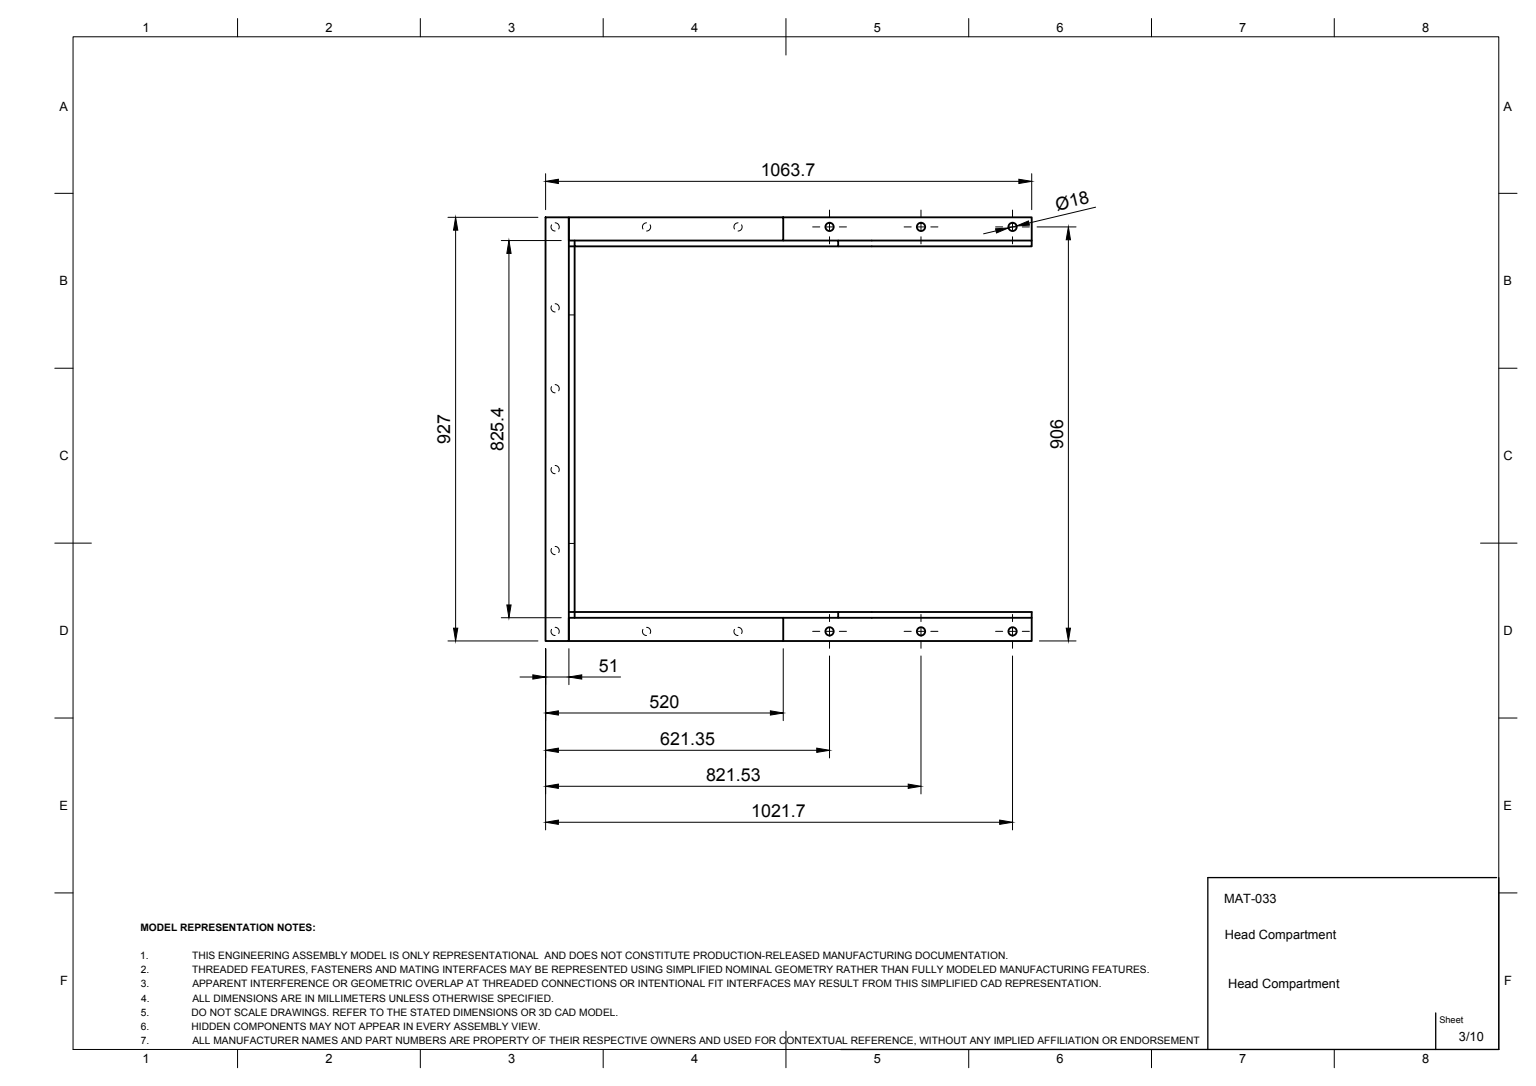
ISO-10303-21;
HEADER;
/* Generated by software containing ST-Developer
 * from STEP Tools, Inc. (www.steptools.com) 
 */

FILE_DESCRIPTION(
/* description */ ('STEP AP214'),
/* implementation_level */ '2;1');

FILE_NAME(
/* name */ 'Head Compartment.step',
/* time_stamp */ '2026-11-14T07:13:32-08:00',
/* author */ (''),
/* organization */ (''),
/* preprocessor_version */ 'ST-DEVELOPER v20.2',
/* originating_system */ 'Autodesk Translation Framework v15.17.0.0',
/* authorisation */ '');

FILE_SCHEMA (('AUTOMOTIVE_DESIGN { 1 0 10303 214 3 1 1 }'));
ENDSEC;

DATA;
#10=MECHANICAL_DESIGN_GEOMETRIC_PRESENTATION_REPRESENTATION('',(#1291,#1292,#1293,#1294,#1295,#1296,#1297,#1298,#1299),#32903);
#672=SHAPE_REPRESENTATION_RELATIONSHIP('SRR','None',#33013,#686);
#686=ADVANCED_BREP_SHAPE_REPRESENTATION('',(#1380,#1381,#1382,#1383,#1384,
#1385,#1386,#1387,#1388),#32888);
#700=CIRCLE('',#15798,75.0000000000001);
#701=CIRCLE('',#15799,75.0000000000001);
#702=CIRCLE('',#15808,75.0000000000001);
#703=CIRCLE('',#15809,75.0000000000001);
#704=CIRCLE('',#15816,8.99999999999998);
#705=CIRCLE('',#15817,8.99999999999998);
#706=CIRCLE('',#15819,8.99999999999998);
#707=CIRCLE('',#15820,8.99999999999998);
#708=CIRCLE('',#15822,8.99999999999998);
#709=CIRCLE('',#15823,8.99999999999998);
#710=CIRCLE('',#15825,8.99999999999998);
#711=CIRCLE('',#15826,8.99999999999998);
#712=CIRCLE('',#15828,8.99999999999998);
#713=CIRCLE('',#15829,8.99999999999998);
#714=CIRCLE('',#15831,8.99999999999998);
#715=CIRCLE('',#15832,8.99999999999998);
#716=CIRCLE('',#15840,8.99999999999998);
#717=CIRCLE('',#15841,8.99999999999998);
#718=CIRCLE('',#15843,9.00000000000001);
#719=CIRCLE('',#15844,9.00000000000001);
#720=CIRCLE('',#15846,9.00000000000001);
#721=CIRCLE('',#15847,9.00000000000001);
#722=CIRCLE('',#15849,9.00000000000001);
#723=CIRCLE('',#15850,9.00000000000001);
#724=CIRCLE('',#15852,9.00000000000001);
#725=CIRCLE('',#15853,9.00000000000001);
#726=CIRCLE('',#15861,8.99999999999998);
#727=CIRCLE('',#15862,8.99999999999998);
#728=CIRCLE('',#15864,9.00000000000001);
#729=CIRCLE('',#15865,9.00000000000001);
#730=CIRCLE('',#15867,9.00000000000001);
#731=CIRCLE('',#15868,9.00000000000001);
#732=CIRCLE('',#15870,9.00000000000001);
#733=CIRCLE('',#15871,9.00000000000001);
#734=CIRCLE('',#15873,9.00000000000001);
#735=CIRCLE('',#15874,9.00000000000001);
#1081=CYLINDRICAL_SURFACE('',#15797,75.0000000000001);
#1082=CYLINDRICAL_SURFACE('',#15807,75.0000000000001);
#1083=CYLINDRICAL_SURFACE('',#15815,8.99999999999998);
#1084=CYLINDRICAL_SURFACE('',#15818,8.99999999999998);
#1085=CYLINDRICAL_SURFACE('',#15821,8.99999999999998);
#1086=CYLINDRICAL_SURFACE('',#15824,8.99999999999998);
#1087=CYLINDRICAL_SURFACE('',#15827,8.99999999999998);
#1088=CYLINDRICAL_SURFACE('',#15830,8.99999999999998);
#1089=CYLINDRICAL_SURFACE('',#15839,8.99999999999998);
#1090=CYLINDRICAL_SURFACE('',#15842,9.00000000000001);
#1091=CYLINDRICAL_SURFACE('',#15845,9.00000000000001);
#1092=CYLINDRICAL_SURFACE('',#15848,9.00000000000001);
#1093=CYLINDRICAL_SURFACE('',#15851,9.00000000000001);
#1094=CYLINDRICAL_SURFACE('',#15860,8.99999999999998);
#1095=CYLINDRICAL_SURFACE('',#15863,9.00000000000001);
#1096=CYLINDRICAL_SURFACE('',#15866,9.00000000000001);
#1097=CYLINDRICAL_SURFACE('',#15869,9.00000000000001);
#1098=CYLINDRICAL_SURFACE('',#15872,9.00000000000001);
#1291=STYLED_ITEM('',(#33097),#1380);
#1292=STYLED_ITEM('',(#33097),#1381);
#1293=STYLED_ITEM('',(#33097),#1382);
#1294=STYLED_ITEM('',(#33097),#1383);
#1295=STYLED_ITEM('',(#33097),#1384);
#1296=STYLED_ITEM('',(#33097),#1385);
#1297=STYLED_ITEM('',(#33097),#1386);
#1298=STYLED_ITEM('',(#33097),#1387);
#1299=STYLED_ITEM('',(#33097),#1388);
#1380=MANIFOLD_SOLID_BREP('Body1',#15539);
#1381=MANIFOLD_SOLID_BREP('Body2',#15540);
#1382=MANIFOLD_SOLID_BREP('Body3',#15541);
#1383=MANIFOLD_SOLID_BREP('Body4',#15542);
#1384=MANIFOLD_SOLID_BREP('Body5',#15543);
#1385=MANIFOLD_SOLID_BREP('Body6',#15544);
#1386=MANIFOLD_SOLID_BREP('Body7',#15545);
#1387=MANIFOLD_SOLID_BREP('Body8',#15546);
#1388=MANIFOLD_SOLID_BREP('Body9',#15547);
#1469=FACE_BOUND('',#2576,.T.);
#1470=FACE_BOUND('',#2578,.T.);
#1471=FACE_BOUND('',#2606,.T.);
#1472=FACE_BOUND('',#2607,.T.);
#1473=FACE_BOUND('',#2608,.T.);
#1474=FACE_BOUND('',#2609,.T.);
#1475=FACE_BOUND('',#2610,.T.);
#1476=FACE_BOUND('',#2611,.T.);
#1477=FACE_BOUND('',#2613,.T.);
#1478=FACE_BOUND('',#2614,.T.);
#1479=FACE_BOUND('',#2615,.T.);
#1480=FACE_BOUND('',#2616,.T.);
#1481=FACE_BOUND('',#2617,.T.);
#1482=FACE_BOUND('',#2618,.T.);
#1483=FACE_BOUND('',#2633,.T.);
#1484=FACE_BOUND('',#2634,.T.);
#1485=FACE_BOUND('',#2635,.T.);
#1486=FACE_BOUND('',#2636,.T.);
#1487=FACE_BOUND('',#2637,.T.);
#1488=FACE_BOUND('',#2639,.T.);
#1489=FACE_BOUND('',#2640,.T.);
#1490=FACE_BOUND('',#2641,.T.);
#1491=FACE_BOUND('',#2642,.T.);
#1492=FACE_BOUND('',#2643,.T.);
#1493=FACE_BOUND('',#2654,.T.);
#1494=FACE_BOUND('',#2655,.T.);
#1495=FACE_BOUND('',#2656,.T.);
#1496=FACE_BOUND('',#2657,.T.);
#1497=FACE_BOUND('',#2658,.T.);
#1498=FACE_BOUND('',#2660,.T.);
#1499=FACE_BOUND('',#2661,.T.);
#1500=FACE_BOUND('',#2662,.T.);
#1501=FACE_BOUND('',#2663,.T.);
#1502=FACE_BOUND('',#2664,.T.);
#1676=FACE_OUTER_BOUND('',#2571,.T.);
#1677=FACE_OUTER_BOUND('',#2572,.T.);
#1678=FACE_OUTER_BOUND('',#2573,.T.);
#1679=FACE_OUTER_BOUND('',#2574,.T.);
#1680=FACE_OUTER_BOUND('',#2575,.T.);
#1681=FACE_OUTER_BOUND('',#2577,.T.);
#1682=FACE_OUTER_BOUND('',#2579,.T.);
#1683=FACE_OUTER_BOUND('',#2580,.T.);
#1684=FACE_OUTER_BOUND('',#2581,.T.);
#1685=FACE_OUTER_BOUND('',#2582,.T.);
#1686=FACE_OUTER_BOUND('',#2583,.T.);
#1687=FACE_OUTER_BOUND('',#2584,.T.);
#1688=FACE_OUTER_BOUND('',#2585,.T.);
#1689=FACE_OUTER_BOUND('',#2586,.T.);
#1690=FACE_OUTER_BOUND('',#2587,.T.);
#1691=FACE_OUTER_BOUND('',#2588,.T.);
#1692=FACE_OUTER_BOUND('',#2589,.T.);
#1693=FACE_OUTER_BOUND('',#2590,.T.);
#1694=FACE_OUTER_BOUND('',#2591,.T.);
#1695=FACE_OUTER_BOUND('',#2592,.T.);
#1696=FACE_OUTER_BOUND('',#2593,.T.);
#1697=FACE_OUTER_BOUND('',#2594,.T.);
#1698=FACE_OUTER_BOUND('',#2595,.T.);
#1699=FACE_OUTER_BOUND('',#2596,.T.);
#1700=FACE_OUTER_BOUND('',#2597,.T.);
#1701=FACE_OUTER_BOUND('',#2598,.T.);
#1702=FACE_OUTER_BOUND('',#2599,.T.);
#1703=FACE_OUTER_BOUND('',#2600,.T.);
#1704=FACE_OUTER_BOUND('',#2601,.T.);
#1705=FACE_OUTER_BOUND('',#2602,.T.);
#1706=FACE_OUTER_BOUND('',#2603,.T.);
#1707=FACE_OUTER_BOUND('',#2604,.T.);
#1708=FACE_OUTER_BOUND('',#2605,.T.);
#1709=FACE_OUTER_BOUND('',#2612,.T.);
#1710=FACE_OUTER_BOUND('',#2619,.T.);
#1711=FACE_OUTER_BOUND('',#2620,.T.);
#1712=FACE_OUTER_BOUND('',#2621,.T.);
#1713=FACE_OUTER_BOUND('',#2622,.T.);
#1714=FACE_OUTER_BOUND('',#2623,.T.);
#1715=FACE_OUTER_BOUND('',#2624,.T.);
#1716=FACE_OUTER_BOUND('',#2625,.T.);
#1717=FACE_OUTER_BOUND('',#2626,.T.);
#1718=FACE_OUTER_BOUND('',#2627,.T.);
#1719=FACE_OUTER_BOUND('',#2628,.T.);
#1720=FACE_OUTER_BOUND('',#2629,.T.);
#1721=FACE_OUTER_BOUND('',#2630,.T.);
#1722=FACE_OUTER_BOUND('',#2631,.T.);
#1723=FACE_OUTER_BOUND('',#2632,.T.);
#1724=FACE_OUTER_BOUND('',#2638,.T.);
#1725=FACE_OUTER_BOUND('',#2644,.T.);
#1726=FACE_OUTER_BOUND('',#2645,.T.);
#1727=FACE_OUTER_BOUND('',#2646,.T.);
#1728=FACE_OUTER_BOUND('',#2647,.T.);
#1729=FACE_OUTER_BOUND('',#2648,.T.);
#1730=FACE_OUTER_BOUND('',#2649,.T.);
#1731=FACE_OUTER_BOUND('',#2650,.T.);
#1732=FACE_OUTER_BOUND('',#2651,.T.);
#1733=FACE_OUTER_BOUND('',#2652,.T.);
#1734=FACE_OUTER_BOUND('',#2653,.T.);
#1735=FACE_OUTER_BOUND('',#2659,.T.);
#1736=FACE_OUTER_BOUND('',#2665,.T.);
#1737=FACE_OUTER_BOUND('',#2666,.T.);
#1738=FACE_OUTER_BOUND('',#2667,.T.);
#1739=FACE_OUTER_BOUND('',#2668,.T.);
#1740=FACE_OUTER_BOUND('',#2669,.T.);
#1741=FACE_OUTER_BOUND('',#2670,.T.);
#1742=FACE_OUTER_BOUND('',#2671,.T.);
#1743=FACE_OUTER_BOUND('',#2672,.T.);
#1744=FACE_OUTER_BOUND('',#2673,.T.);
#1745=FACE_OUTER_BOUND('',#2674,.T.);
#1746=FACE_OUTER_BOUND('',#2675,.T.);
#1747=FACE_OUTER_BOUND('',#2676,.T.);
#1748=FACE_OUTER_BOUND('',#2677,.T.);
#1749=FACE_OUTER_BOUND('',#2678,.T.);
#1750=FACE_OUTER_BOUND('',#2679,.T.);
#1751=FACE_OUTER_BOUND('',#2680,.T.);
#1752=FACE_OUTER_BOUND('',#2681,.T.);
#1753=FACE_OUTER_BOUND('',#2682,.T.);
#2571=EDGE_LOOP('',(#9907,#9908,#9909,#9910));
#2572=EDGE_LOOP('',(#9911,#9912,#9913,#9914));
#2573=EDGE_LOOP('',(#9915,#9916,#9917,#9918));
#2574=EDGE_LOOP('',(#9919,#9920,#9921,#9922));
#2575=EDGE_LOOP('',(#9923,#9924,#9925,#9926));
#2576=EDGE_LOOP('',(#9927,#9928,#9929,#9930));
#2577=EDGE_LOOP('',(#9931,#9932,#9933,#9934));
#2578=EDGE_LOOP('',(#9935,#9936,#9937,#9938));
#2579=EDGE_LOOP('',(#9939,#9940,#9941,#9942));
#2580=EDGE_LOOP('',(#9943,#9944,#9945,#9946));
#2581=EDGE_LOOP('',(#9947,#9948,#9949,#9950));
#2582=EDGE_LOOP('',(#9951,#9952,#9953,#9954));
#2583=EDGE_LOOP('',(#9955,#9956,#9957,#9958));
#2584=EDGE_LOOP('',(#9959,#9960,#9961,#9962));
#2585=EDGE_LOOP('',(#9963,#9964,#9965,#9966));
#2586=EDGE_LOOP('',(#9967,#9968,#9969,#9970));
#2587=EDGE_LOOP('',(#9971,#9972,#9973,#9974));
#2588=EDGE_LOOP('',(#9975,#9976,#9977,#9978));
#2589=EDGE_LOOP('',(#9979,#9980,#9981,#9982,#9983,#9984));
#2590=EDGE_LOOP('',(#9985,#9986,#9987,#9988,#9989,#9990));
#2591=EDGE_LOOP('',(#9991,#9992,#9993,#9994));
#2592=EDGE_LOOP('',(#9995,#9996,#9997,#9998));
#2593=EDGE_LOOP('',(#9999,#10000,#10001,#10002));
#2594=EDGE_LOOP('',(#10003,#10004,#10005,#10006));
#2595=EDGE_LOOP('',(#10007,#10008,#10009,#10010));
#2596=EDGE_LOOP('',(#10011,#10012,#10013,#10014));
#2597=EDGE_LOOP('',(#10015,#10016,#10017,#10018,#10019,#10020));
#2598=EDGE_LOOP('',(#10021,#10022,#10023,#10024,#10025,#10026));
#2599=EDGE_LOOP('',(#10027,#10028,#10029,#10030));
#2600=EDGE_LOOP('',(#10031,#10032,#10033,#10034));
#2601=EDGE_LOOP('',(#10035,#10036,#10037,#10038));
#2602=EDGE_LOOP('',(#10039,#10040,#10041,#10042));
#2603=EDGE_LOOP('',(#10043,#10044,#10045,#10046));
#2604=EDGE_LOOP('',(#10047,#10048,#10049,#10050));
#2605=EDGE_LOOP('',(#10051,#10052,#10053,#10054));
#2606=EDGE_LOOP('',(#10055));
#2607=EDGE_LOOP('',(#10056));
#2608=EDGE_LOOP('',(#10057));
#2609=EDGE_LOOP('',(#10058));
#2610=EDGE_LOOP('',(#10059));
#2611=EDGE_LOOP('',(#10060));
#2612=EDGE_LOOP('',(#10061,#10062,#10063,#10064));
#2613=EDGE_LOOP('',(#10065));
#2614=EDGE_LOOP('',(#10066));
#2615=EDGE_LOOP('',(#10067));
#2616=EDGE_LOOP('',(#10068));
#2617=EDGE_LOOP('',(#10069));
#2618=EDGE_LOOP('',(#10070));
#2619=EDGE_LOOP('',(#10071,#10072,#10073,#10074));
#2620=EDGE_LOOP('',(#10075,#10076,#10077,#10078));
#2621=EDGE_LOOP('',(#10079,#10080,#10081,#10082));
#2622=EDGE_LOOP('',(#10083,#10084,#10085,#10086));
#2623=EDGE_LOOP('',(#10087,#10088,#10089,#10090));
#2624=EDGE_LOOP('',(#10091,#10092,#10093,#10094));
#2625=EDGE_LOOP('',(#10095,#10096,#10097,#10098));
#2626=EDGE_LOOP('',(#10099,#10100,#10101,#10102));
#2627=EDGE_LOOP('',(#10103,#10104,#10105,#10106));
#2628=EDGE_LOOP('',(#10107,#10108,#10109,#10110));
#2629=EDGE_LOOP('',(#10111,#10112,#10113,#10114));
#2630=EDGE_LOOP('',(#10115,#10116,#10117,#10118));
#2631=EDGE_LOOP('',(#10119,#10120,#10121,#10122));
#2632=EDGE_LOOP('',(#10123,#10124,#10125,#10126));
#2633=EDGE_LOOP('',(#10127));
#2634=EDGE_LOOP('',(#10128));
#2635=EDGE_LOOP('',(#10129));
#2636=EDGE_LOOP('',(#10130));
#2637=EDGE_LOOP('',(#10131));
#2638=EDGE_LOOP('',(#10132,#10133,#10134,#10135));
#2639=EDGE_LOOP('',(#10136));
#2640=EDGE_LOOP('',(#10137));
#2641=EDGE_LOOP('',(#10138));
#2642=EDGE_LOOP('',(#10139));
#2643=EDGE_LOOP('',(#10140));
#2644=EDGE_LOOP('',(#10141,#10142,#10143,#10144));
#2645=EDGE_LOOP('',(#10145,#10146,#10147,#10148));
#2646=EDGE_LOOP('',(#10149,#10150,#10151,#10152));
#2647=EDGE_LOOP('',(#10153,#10154,#10155,#10156));
#2648=EDGE_LOOP('',(#10157,#10158,#10159,#10160));
#2649=EDGE_LOOP('',(#10161,#10162,#10163,#10164));
#2650=EDGE_LOOP('',(#10165,#10166,#10167,#10168));
#2651=EDGE_LOOP('',(#10169,#10170,#10171,#10172));
#2652=EDGE_LOOP('',(#10173,#10174,#10175,#10176));
#2653=EDGE_LOOP('',(#10177,#10178,#10179,#10180));
#2654=EDGE_LOOP('',(#10181));
#2655=EDGE_LOOP('',(#10182));
#2656=EDGE_LOOP('',(#10183));
#2657=EDGE_LOOP('',(#10184));
#2658=EDGE_LOOP('',(#10185));
#2659=EDGE_LOOP('',(#10186,#10187,#10188,#10189));
#2660=EDGE_LOOP('',(#10190));
#2661=EDGE_LOOP('',(#10191));
#2662=EDGE_LOOP('',(#10192));
#2663=EDGE_LOOP('',(#10193));
#2664=EDGE_LOOP('',(#10194));
#2665=EDGE_LOOP('',(#10195,#10196,#10197,#10198));
#2666=EDGE_LOOP('',(#10199,#10200,#10201,#10202));
#2667=EDGE_LOOP('',(#10203,#10204,#10205,#10206));
#2668=EDGE_LOOP('',(#10207,#10208,#10209,#10210));
#2669=EDGE_LOOP('',(#10211,#10212,#10213,#10214));
#2670=EDGE_LOOP('',(#10215,#10216,#10217,#10218));
#2671=EDGE_LOOP('',(#10219,#10220,#10221,#10222));
#2672=EDGE_LOOP('',(#10223,#10224,#10225,#10226));
#2673=EDGE_LOOP('',(#10227,#10228,#10229,#10230));
#2674=EDGE_LOOP('',(#10231,#10232,#10233,#10234));
#2675=EDGE_LOOP('',(#10235,#10236,#10237,#10238));
#2676=EDGE_LOOP('',(#10239,#10240,#10241,#10242));
#2677=EDGE_LOOP('',(#10243,#10244,#10245,#10246));
#2678=EDGE_LOOP('',(#10247,#10248,#10249,#10250));
#2679=EDGE_LOOP('',(#10251,#10252,#10253,#10254));
#2680=EDGE_LOOP('',(#10255,#10256,#10257,#10258));
#2681=EDGE_LOOP('',(#10259,#10260,#10261,#10262));
#2682=EDGE_LOOP('',(#10263,#10264,#10265,#10266));
#3673=LINE('',#21314,#5077);
#3674=LINE('',#21316,#5078);
#3675=LINE('',#21318,#5079);
#3676=LINE('',#21319,#5080);
#3677=LINE('',#21322,#5081);
#3678=LINE('',#21324,#5082);
#3679=LINE('',#21325,#5083);
#3680=LINE('',#21328,#5084);
#3681=LINE('',#21330,#5085);
#3682=LINE('',#21331,#5086);
#3683=LINE('',#21333,#5087);
#3684=LINE('',#21334,#5088);
#3685=LINE('',#21338,#5089);
#3686=LINE('',#21340,#5090);
#3687=LINE('',#21342,#5091);
#3688=LINE('',#21343,#5092);
#3689=LINE('',#21347,#5093);
#3690=LINE('',#21349,#5094);
#3691=LINE('',#21351,#5095);
#3692=LINE('',#21352,#5096);
#3693=LINE('',#21354,#5097);
#3694=LINE('',#21355,#5098);
#3695=LINE('',#21357,#5099);
#3696=LINE('',#21359,#5100);
#3697=LINE('',#21364,#5101);
#3698=LINE('',#21366,#5102);
#3699=LINE('',#21368,#5103);
#3700=LINE('',#21369,#5104);
#3701=LINE('',#21372,#5105);
#3702=LINE('',#21374,#5106);
#3703=LINE('',#21375,#5107);
#3704=LINE('',#21380,#5108);
#3705=LINE('',#21384,#5109);
#3706=LINE('',#21386,#5110);
#3707=LINE('',#21387,#5111);
#3708=LINE('',#21390,#5112);
#3709=LINE('',#21392,#5113);
#3710=LINE('',#21393,#5114);
#3711=LINE('',#21395,#5115);
#3712=LINE('',#21396,#5116);
#3713=LINE('',#21402,#5117);
#3714=LINE('',#21404,#5118);
#3715=LINE('',#21406,#5119);
#3716=LINE('',#21407,#5120);
#3717=LINE('',#21410,#5121);
#3718=LINE('',#21412,#5122);
#3719=LINE('',#21413,#5123);
#3720=LINE('',#21419,#5124);
#3721=LINE('',#21422,#5125);
#3722=LINE('',#21424,#5126);
#3723=LINE('',#21425,#5127);
#3724=LINE('',#21428,#5128);
#3725=LINE('',#21430,#5129);
#3726=LINE('',#21431,#5130);
#3727=LINE('',#21433,#5131);
#3728=LINE('',#21434,#5132);
#3729=LINE('',#21441,#5133);
#3730=LINE('',#21447,#5134);
#3731=LINE('',#21453,#5135);
#3732=LINE('',#21459,#5136);
#3733=LINE('',#21465,#5137);
#3734=LINE('',#21471,#5138);
#3735=LINE('',#21476,#5139);
#3736=LINE('',#21478,#5140);
#3737=LINE('',#21480,#5141);
#3738=LINE('',#21481,#5142);
#3739=LINE('',#21485,#5143);
#3740=LINE('',#21487,#5144);
#3741=LINE('',#21489,#5145);
#3742=LINE('',#21490,#5146);
#3743=LINE('',#21492,#5147);
#3744=LINE('',#21493,#5148);
#3745=LINE('',#21495,#5149);
#3746=LINE('',#21497,#5150);
#3747=LINE('',#21503,#5151);
#3748=LINE('',#21509,#5152);
#3749=LINE('',#21515,#5153);
#3750=LINE('',#21521,#5154);
#3751=LINE('',#21527,#5155);
#3752=LINE('',#21532,#5156);
#3753=LINE('',#21534,#5157);
#3754=LINE('',#21536,#5158);
#3755=LINE('',#21537,#5159);
#3756=LINE('',#21540,#5160);
#3757=LINE('',#21542,#5161);
#3758=LINE('',#21543,#5162);
#3759=LINE('',#21546,#5163);
#3760=LINE('',#21548,#5164);
#3761=LINE('',#21549,#5165);
#3762=LINE('',#21551,#5166);
#3763=LINE('',#21552,#5167);
#3764=LINE('',#21559,#5168);
#3765=LINE('',#21565,#5169);
#3766=LINE('',#21571,#5170);
#3767=LINE('',#21577,#5171);
#3768=LINE('',#21583,#5172);
#3769=LINE('',#21588,#5173);
#3770=LINE('',#21590,#5174);
#3771=LINE('',#21592,#5175);
#3772=LINE('',#21593,#5176);
#3773=LINE('',#21596,#5177);
#3774=LINE('',#21598,#5178);
#3775=LINE('',#21599,#5179);
#3776=LINE('',#21602,#5180);
#3777=LINE('',#21604,#5181);
#3778=LINE('',#21605,#5182);
#3779=LINE('',#21607,#5183);
#3780=LINE('',#21608,#5184);
#3781=LINE('',#21614,#5185);
#3782=LINE('',#21616,#5186);
#3783=LINE('',#21618,#5187);
#3784=LINE('',#21619,#5188);
#3785=LINE('',#21622,#5189);
#3786=LINE('',#21624,#5190);
#3787=LINE('',#21625,#5191);
#3788=LINE('',#21628,#5192);
#3789=LINE('',#21630,#5193);
#3790=LINE('',#21631,#5194);
#3791=LINE('',#21633,#5195);
#3792=LINE('',#21634,#5196);
#3793=LINE('',#21640,#5197);
#3794=LINE('',#21642,#5198);
#3795=LINE('',#21644,#5199);
#3796=LINE('',#21645,#5200);
#3797=LINE('',#21648,#5201);
#3798=LINE('',#21650,#5202);
#3799=LINE('',#21651,#5203);
#3800=LINE('',#21654,#5204);
#3801=LINE('',#21656,#5205);
#3802=LINE('',#21657,#5206);
#3803=LINE('',#21659,#5207);
#3804=LINE('',#21660,#5208);
#3805=LINE('',#21666,#5209);
#3806=LINE('',#21668,#5210);
#3807=LINE('',#21670,#5211);
#3808=LINE('',#21671,#5212);
#3809=LINE('',#21674,#5213);
#3810=LINE('',#21676,#5214);
#3811=LINE('',#21677,#5215);
#3812=LINE('',#21680,#5216);
#3813=LINE('',#21682,#5217);
#3814=LINE('',#21683,#5218);
#3815=LINE('',#21685,#5219);
#3816=LINE('',#21686,#5220);
#5077=VECTOR('',#17163,1000.);
#5078=VECTOR('',#17164,1000.);
#5079=VECTOR('',#17165,1000.);
#5080=VECTOR('',#17166,1000.);
#5081=VECTOR('',#17169,1000.);
#5082=VECTOR('',#17170,1000.);
#5083=VECTOR('',#17171,1000.);
#5084=VECTOR('',#17174,1000.);
#5085=VECTOR('',#17175,1000.);
#5086=VECTOR('',#17176,1000.);
#5087=VECTOR('',#17179,1000.);
#5088=VECTOR('',#17180,1000.);
#5089=VECTOR('',#17183,1000.);
#5090=VECTOR('',#17184,1000.);
#5091=VECTOR('',#17185,1000.);
#5092=VECTOR('',#17186,1000.);
#5093=VECTOR('',#17189,1000.);
#5094=VECTOR('',#17190,1000.);
#5095=VECTOR('',#17191,1000.);
#5096=VECTOR('',#17192,1000.);
#5097=VECTOR('',#17195,1000.);
#5098=VECTOR('',#17196,1000.);
#5099=VECTOR('',#17199,1000.);
#5100=VECTOR('',#17202,1000.);
#5101=VECTOR('',#17207,1000.);
#5102=VECTOR('',#17208,1000.);
#5103=VECTOR('',#17209,1000.);
#5104=VECTOR('',#17210,1000.);
#5105=VECTOR('',#17213,1000.);
#5106=VECTOR('',#17214,1000.);
#5107=VECTOR('',#17215,1000.);
#5108=VECTOR('',#17220,1000.);
#5109=VECTOR('',#17225,1000.);
#5110=VECTOR('',#17226,1000.);
#5111=VECTOR('',#17227,1000.);
#5112=VECTOR('',#17230,1000.);
#5113=VECTOR('',#17231,1000.);
#5114=VECTOR('',#17232,1000.);
#5115=VECTOR('',#17235,1000.);
#5116=VECTOR('',#17236,1000.);
#5117=VECTOR('',#17243,1000.);
#5118=VECTOR('',#17244,1000.);
#5119=VECTOR('',#17245,1000.);
#5120=VECTOR('',#17246,1000.);
#5121=VECTOR('',#17249,1000.);
#5122=VECTOR('',#17250,1000.);
#5123=VECTOR('',#17251,1000.);
#5124=VECTOR('',#17258,1000.);
#5125=VECTOR('',#17261,1000.);
#5126=VECTOR('',#17262,1000.);
#5127=VECTOR('',#17263,1000.);
#5128=VECTOR('',#17266,1000.);
#5129=VECTOR('',#17267,1000.);
#5130=VECTOR('',#17268,1000.);
#5131=VECTOR('',#17271,1000.);
#5132=VECTOR('',#17272,1000.);
#5133=VECTOR('',#17281,8.99999999999998);
#5134=VECTOR('',#17288,8.99999999999998);
#5135=VECTOR('',#17295,8.99999999999998);
#5136=VECTOR('',#17302,8.99999999999998);
#5137=VECTOR('',#17309,8.99999999999998);
#5138=VECTOR('',#17316,8.99999999999998);
#5139=VECTOR('',#17321,1000.);
#5140=VECTOR('',#17322,1000.);
#5141=VECTOR('',#17323,1000.);
#5142=VECTOR('',#17324,1000.);
#5143=VECTOR('',#17327,1000.);
#5144=VECTOR('',#17328,1000.);
#5145=VECTOR('',#17329,1000.);
#5146=VECTOR('',#17330,1000.);
#5147=VECTOR('',#17333,1000.);
#5148=VECTOR('',#17334,1000.);
#5149=VECTOR('',#17337,1000.);
#5150=VECTOR('',#17340,1000.);
#5151=VECTOR('',#17347,8.99999999999998);
#5152=VECTOR('',#17354,9.00000000000001);
#5153=VECTOR('',#17361,9.00000000000001);
#5154=VECTOR('',#17368,9.00000000000001);
#5155=VECTOR('',#17375,9.00000000000001);
#5156=VECTOR('',#17380,1000.);
#5157=VECTOR('',#17381,1000.);
#5158=VECTOR('',#17382,1000.);
#5159=VECTOR('',#17383,1000.);
#5160=VECTOR('',#17386,1000.);
#5161=VECTOR('',#17387,1000.);
#5162=VECTOR('',#17388,1000.);
#5163=VECTOR('',#17391,1000.);
#5164=VECTOR('',#17392,1000.);
#5165=VECTOR('',#17393,1000.);
#5166=VECTOR('',#17396,1000.);
#5167=VECTOR('',#17397,1000.);
#5168=VECTOR('',#17406,8.99999999999998);
#5169=VECTOR('',#17413,9.00000000000001);
#5170=VECTOR('',#17420,9.00000000000001);
#5171=VECTOR('',#17427,9.00000000000001);
#5172=VECTOR('',#17434,9.00000000000001);
#5173=VECTOR('',#17439,1000.);
#5174=VECTOR('',#17440,1000.);
#5175=VECTOR('',#17441,1000.);
#5176=VECTOR('',#17442,1000.);
#5177=VECTOR('',#17445,1000.);
#5178=VECTOR('',#17446,1000.);
#5179=VECTOR('',#17447,1000.);
#5180=VECTOR('',#17450,1000.);
#5181=VECTOR('',#17451,1000.);
#5182=VECTOR('',#17452,1000.);
#5183=VECTOR('',#17455,1000.);
#5184=VECTOR('',#17456,1000.);
#5185=VECTOR('',#17463,1000.);
#5186=VECTOR('',#17464,1000.);
#5187=VECTOR('',#17465,1000.);
#5188=VECTOR('',#17466,1000.);
#5189=VECTOR('',#17469,1000.);
#5190=VECTOR('',#17470,1000.);
#5191=VECTOR('',#17471,1000.);
#5192=VECTOR('',#17474,1000.);
#5193=VECTOR('',#17475,1000.);
#5194=VECTOR('',#17476,1000.);
#5195=VECTOR('',#17479,1000.);
#5196=VECTOR('',#17480,1000.);
#5197=VECTOR('',#17487,1000.);
#5198=VECTOR('',#17488,1000.);
#5199=VECTOR('',#17489,1000.);
#5200=VECTOR('',#17490,1000.);
#5201=VECTOR('',#17493,1000.);
#5202=VECTOR('',#17494,1000.);
#5203=VECTOR('',#17495,1000.);
#5204=VECTOR('',#17498,1000.);
#5205=VECTOR('',#17499,1000.);
#5206=VECTOR('',#17500,1000.);
#5207=VECTOR('',#17503,1000.);
#5208=VECTOR('',#17504,1000.);
#5209=VECTOR('',#17511,1000.);
#5210=VECTOR('',#17512,1000.);
#5211=VECTOR('',#17513,1000.);
#5212=VECTOR('',#17514,1000.);
#5213=VECTOR('',#17517,1000.);
#5214=VECTOR('',#17518,1000.);
#5215=VECTOR('',#17519,1000.);
#5216=VECTOR('',#17522,1000.);
#5217=VECTOR('',#17523,1000.);
#5218=VECTOR('',#17524,1000.);
#5219=VECTOR('',#17527,1000.);
#5220=VECTOR('',#17528,1000.);
#6481=VERTEX_POINT('',#21312);
#6482=VERTEX_POINT('',#21313);
#6483=VERTEX_POINT('',#21315);
#6484=VERTEX_POINT('',#21317);
#6485=VERTEX_POINT('',#21321);
#6486=VERTEX_POINT('',#21323);
#6487=VERTEX_POINT('',#21327);
#6488=VERTEX_POINT('',#21329);
#6489=VERTEX_POINT('',#21336);
#6490=VERTEX_POINT('',#21337);
#6491=VERTEX_POINT('',#21339);
#6492=VERTEX_POINT('',#21341);
#6493=VERTEX_POINT('',#21345);
#6494=VERTEX_POINT('',#21346);
#6495=VERTEX_POINT('',#21348);
#6496=VERTEX_POINT('',#21350);
#6497=VERTEX_POINT('',#21362);
#6498=VERTEX_POINT('',#21363);
#6499=VERTEX_POINT('',#21365);
#6500=VERTEX_POINT('',#21367);
#6501=VERTEX_POINT('',#21371);
#6502=VERTEX_POINT('',#21373);
#6503=VERTEX_POINT('',#21377);
#6504=VERTEX_POINT('',#21379);
#6505=VERTEX_POINT('',#21383);
#6506=VERTEX_POINT('',#21385);
#6507=VERTEX_POINT('',#21389);
#6508=VERTEX_POINT('',#21391);
#6509=VERTEX_POINT('',#21400);
#6510=VERTEX_POINT('',#21401);
#6511=VERTEX_POINT('',#21403);
#6512=VERTEX_POINT('',#21405);
#6513=VERTEX_POINT('',#21409);
#6514=VERTEX_POINT('',#21411);
#6515=VERTEX_POINT('',#21415);
#6516=VERTEX_POINT('',#21417);
#6517=VERTEX_POINT('',#21421);
#6518=VERTEX_POINT('',#21423);
#6519=VERTEX_POINT('',#21427);
#6520=VERTEX_POINT('',#21429);
#6521=VERTEX_POINT('',#21438);
#6522=VERTEX_POINT('',#21440);
#6523=VERTEX_POINT('',#21444);
#6524=VERTEX_POINT('',#21446);
#6525=VERTEX_POINT('',#21450);
#6526=VERTEX_POINT('',#21452);
#6527=VERTEX_POINT('',#21456);
#6528=VERTEX_POINT('',#21458);
#6529=VERTEX_POINT('',#21462);
#6530=VERTEX_POINT('',#21464);
#6531=VERTEX_POINT('',#21468);
#6532=VERTEX_POINT('',#21470);
#6533=VERTEX_POINT('',#21474);
#6534=VERTEX_POINT('',#21475);
#6535=VERTEX_POINT('',#21477);
#6536=VERTEX_POINT('',#21479);
#6537=VERTEX_POINT('',#21483);
#6538=VERTEX_POINT('',#21484);
#6539=VERTEX_POINT('',#21486);
#6540=VERTEX_POINT('',#21488);
#6541=VERTEX_POINT('',#21500);
#6542=VERTEX_POINT('',#21502);
#6543=VERTEX_POINT('',#21506);
#6544=VERTEX_POINT('',#21508);
#6545=VERTEX_POINT('',#21512);
#6546=VERTEX_POINT('',#21514);
#6547=VERTEX_POINT('',#21518);
#6548=VERTEX_POINT('',#21520);
#6549=VERTEX_POINT('',#21524);
#6550=VERTEX_POINT('',#21526);
#6551=VERTEX_POINT('',#21530);
#6552=VERTEX_POINT('',#21531);
#6553=VERTEX_POINT('',#21533);
#6554=VERTEX_POINT('',#21535);
#6555=VERTEX_POINT('',#21539);
#6556=VERTEX_POINT('',#21541);
#6557=VERTEX_POINT('',#21545);
#6558=VERTEX_POINT('',#21547);
#6559=VERTEX_POINT('',#21556);
#6560=VERTEX_POINT('',#21558);
#6561=VERTEX_POINT('',#21562);
#6562=VERTEX_POINT('',#21564);
#6563=VERTEX_POINT('',#21568);
#6564=VERTEX_POINT('',#21570);
#6565=VERTEX_POINT('',#21574);
#6566=VERTEX_POINT('',#21576);
#6567=VERTEX_POINT('',#21580);
#6568=VERTEX_POINT('',#21582);
#6569=VERTEX_POINT('',#21586);
#6570=VERTEX_POINT('',#21587);
#6571=VERTEX_POINT('',#21589);
#6572=VERTEX_POINT('',#21591);
#6573=VERTEX_POINT('',#21595);
#6574=VERTEX_POINT('',#21597);
#6575=VERTEX_POINT('',#21601);
#6576=VERTEX_POINT('',#21603);
#6577=VERTEX_POINT('',#21612);
#6578=VERTEX_POINT('',#21613);
#6579=VERTEX_POINT('',#21615);
#6580=VERTEX_POINT('',#21617);
#6581=VERTEX_POINT('',#21621);
#6582=VERTEX_POINT('',#21623);
#6583=VERTEX_POINT('',#21627);
#6584=VERTEX_POINT('',#21629);
#6585=VERTEX_POINT('',#21638);
#6586=VERTEX_POINT('',#21639);
#6587=VERTEX_POINT('',#21641);
#6588=VERTEX_POINT('',#21643);
#6589=VERTEX_POINT('',#21647);
#6590=VERTEX_POINT('',#21649);
#6591=VERTEX_POINT('',#21653);
#6592=VERTEX_POINT('',#21655);
#6593=VERTEX_POINT('',#21664);
#6594=VERTEX_POINT('',#21665);
#6595=VERTEX_POINT('',#21667);
#6596=VERTEX_POINT('',#21669);
#6597=VERTEX_POINT('',#21673);
#6598=VERTEX_POINT('',#21675);
#6599=VERTEX_POINT('',#21679);
#6600=VERTEX_POINT('',#21681);
#7837=EDGE_CURVE('',#6481,#6482,#3673,.T.);
#7838=EDGE_CURVE('',#6483,#6481,#3674,.T.);
#7839=EDGE_CURVE('',#6483,#6484,#3675,.T.);
#7840=EDGE_CURVE('',#6484,#6482,#3676,.T.);
#7841=EDGE_CURVE('',#6485,#6481,#3677,.T.);
#7842=EDGE_CURVE('',#6486,#6485,#3678,.T.);
#7843=EDGE_CURVE('',#6486,#6483,#3679,.T.);
#7844=EDGE_CURVE('',#6487,#6485,#3680,.T.);
#7845=EDGE_CURVE('',#6488,#6487,#3681,.T.);
#7846=EDGE_CURVE('',#6488,#6486,#3682,.T.);
#7847=EDGE_CURVE('',#6482,#6487,#3683,.T.);
#7848=EDGE_CURVE('',#6484,#6488,#3684,.T.);
#7849=EDGE_CURVE('',#6489,#6490,#3685,.T.);
#7850=EDGE_CURVE('',#6490,#6491,#3686,.T.);
#7851=EDGE_CURVE('',#6491,#6492,#3687,.T.);
#7852=EDGE_CURVE('',#6492,#6489,#3688,.T.);
#7853=EDGE_CURVE('',#6493,#6494,#3689,.T.);
#7854=EDGE_CURVE('',#6495,#6493,#3690,.T.);
#7855=EDGE_CURVE('',#6496,#6495,#3691,.T.);
#7856=EDGE_CURVE('',#6494,#6496,#3692,.T.);
#7857=EDGE_CURVE('',#6490,#6493,#3693,.T.);
#7858=EDGE_CURVE('',#6489,#6495,#3694,.T.);
#7859=EDGE_CURVE('',#6492,#6496,#3695,.T.);
#7860=EDGE_CURVE('',#6491,#6494,#3696,.T.);
#7861=EDGE_CURVE('',#6497,#6498,#3697,.T.);
#7862=EDGE_CURVE('',#6499,#6498,#3698,.T.);
#7863=EDGE_CURVE('',#6500,#6499,#3699,.T.);
#7864=EDGE_CURVE('',#6500,#6497,#3700,.T.);
#7865=EDGE_CURVE('',#6498,#6501,#3701,.T.);
#7866=EDGE_CURVE('',#6502,#6501,#3702,.T.);
#7867=EDGE_CURVE('',#6499,#6502,#3703,.T.);
#7868=EDGE_CURVE('',#6501,#6503,#700,.T.);
#7869=EDGE_CURVE('',#6504,#6503,#3704,.T.);
#7870=EDGE_CURVE('',#6502,#6504,#701,.T.);
#7871=EDGE_CURVE('',#6503,#6505,#3705,.T.);
#7872=EDGE_CURVE('',#6506,#6505,#3706,.T.);
#7873=EDGE_CURVE('',#6504,#6506,#3707,.T.);
#7874=EDGE_CURVE('',#6505,#6507,#3708,.T.);
#7875=EDGE_CURVE('',#6508,#6507,#3709,.T.);
#7876=EDGE_CURVE('',#6506,#6508,#3710,.T.);
#7877=EDGE_CURVE('',#6507,#6497,#3711,.T.);
#7878=EDGE_CURVE('',#6508,#6500,#3712,.T.);
#7879=EDGE_CURVE('',#6509,#6510,#3713,.T.);
#7880=EDGE_CURVE('',#6511,#6509,#3714,.T.);
#7881=EDGE_CURVE('',#6511,#6512,#3715,.T.);
#7882=EDGE_CURVE('',#6512,#6510,#3716,.T.);
#7883=EDGE_CURVE('',#6510,#6513,#3717,.T.);
#7884=EDGE_CURVE('',#6512,#6514,#3718,.T.);
#7885=EDGE_CURVE('',#6514,#6513,#3719,.T.);
#7886=EDGE_CURVE('',#6513,#6515,#702,.T.);
#7887=EDGE_CURVE('',#6514,#6516,#703,.T.);
#7888=EDGE_CURVE('',#6516,#6515,#3720,.T.);
#7889=EDGE_CURVE('',#6515,#6517,#3721,.T.);
#7890=EDGE_CURVE('',#6516,#6518,#3722,.T.);
#7891=EDGE_CURVE('',#6518,#6517,#3723,.T.);
#7892=EDGE_CURVE('',#6517,#6519,#3724,.T.);
#7893=EDGE_CURVE('',#6518,#6520,#3725,.T.);
#7894=EDGE_CURVE('',#6520,#6519,#3726,.T.);
#7895=EDGE_CURVE('',#6519,#6509,#3727,.T.);
#7896=EDGE_CURVE('',#6520,#6511,#3728,.T.);
#7897=EDGE_CURVE('',#6521,#6521,#704,.T.);
#7898=EDGE_CURVE('',#6521,#6522,#3729,.T.);
#7899=EDGE_CURVE('',#6522,#6522,#705,.T.);
#7900=EDGE_CURVE('',#6523,#6523,#706,.T.);
#7901=EDGE_CURVE('',#6523,#6524,#3730,.T.);
#7902=EDGE_CURVE('',#6524,#6524,#707,.T.);
#7903=EDGE_CURVE('',#6525,#6525,#708,.T.);
#7904=EDGE_CURVE('',#6525,#6526,#3731,.T.);
#7905=EDGE_CURVE('',#6526,#6526,#709,.T.);
#7906=EDGE_CURVE('',#6527,#6527,#710,.T.);
#7907=EDGE_CURVE('',#6527,#6528,#3732,.T.);
#7908=EDGE_CURVE('',#6528,#6528,#711,.T.);
#7909=EDGE_CURVE('',#6529,#6529,#712,.T.);
#7910=EDGE_CURVE('',#6529,#6530,#3733,.T.);
#7911=EDGE_CURVE('',#6530,#6530,#713,.T.);
#7912=EDGE_CURVE('',#6531,#6531,#714,.T.);
#7913=EDGE_CURVE('',#6531,#6532,#3734,.T.);
#7914=EDGE_CURVE('',#6532,#6532,#715,.T.);
#7915=EDGE_CURVE('',#6533,#6534,#3735,.T.);
#7916=EDGE_CURVE('',#6534,#6535,#3736,.T.);
#7917=EDGE_CURVE('',#6535,#6536,#3737,.T.);
#7918=EDGE_CURVE('',#6536,#6533,#3738,.T.);
#7919=EDGE_CURVE('',#6537,#6538,#3739,.T.);
#7920=EDGE_CURVE('',#6539,#6537,#3740,.T.);
#7921=EDGE_CURVE('',#6540,#6539,#3741,.T.);
#7922=EDGE_CURVE('',#6538,#6540,#3742,.T.);
#7923=EDGE_CURVE('',#6534,#6538,#3743,.T.);
#7924=EDGE_CURVE('',#6533,#6537,#3744,.T.);
#7925=EDGE_CURVE('',#6535,#6540,#3745,.T.);
#7926=EDGE_CURVE('',#6536,#6539,#3746,.T.);
#7927=EDGE_CURVE('',#6541,#6541,#716,.T.);
#7928=EDGE_CURVE('',#6541,#6542,#3747,.T.);
#7929=EDGE_CURVE('',#6542,#6542,#717,.T.);
#7930=EDGE_CURVE('',#6543,#6543,#718,.T.);
#7931=EDGE_CURVE('',#6543,#6544,#3748,.T.);
#7932=EDGE_CURVE('',#6544,#6544,#719,.T.);
#7933=EDGE_CURVE('',#6545,#6545,#720,.T.);
#7934=EDGE_CURVE('',#6545,#6546,#3749,.T.);
#7935=EDGE_CURVE('',#6546,#6546,#721,.T.);
#7936=EDGE_CURVE('',#6547,#6547,#722,.T.);
#7937=EDGE_CURVE('',#6547,#6548,#3750,.T.);
#7938=EDGE_CURVE('',#6548,#6548,#723,.T.);
#7939=EDGE_CURVE('',#6549,#6549,#724,.T.);
#7940=EDGE_CURVE('',#6549,#6550,#3751,.T.);
#7941=EDGE_CURVE('',#6550,#6550,#725,.T.);
#7942=EDGE_CURVE('',#6551,#6552,#3752,.T.);
#7943=EDGE_CURVE('',#6553,#6551,#3753,.T.);
#7944=EDGE_CURVE('',#6553,#6554,#3754,.T.);
#7945=EDGE_CURVE('',#6554,#6552,#3755,.T.);
#7946=EDGE_CURVE('',#6555,#6551,#3756,.T.);
#7947=EDGE_CURVE('',#6556,#6555,#3757,.T.);
#7948=EDGE_CURVE('',#6556,#6553,#3758,.T.);
#7949=EDGE_CURVE('',#6557,#6555,#3759,.T.);
#7950=EDGE_CURVE('',#6558,#6557,#3760,.T.);
#7951=EDGE_CURVE('',#6558,#6556,#3761,.T.);
#7952=EDGE_CURVE('',#6552,#6557,#3762,.T.);
#7953=EDGE_CURVE('',#6554,#6558,#3763,.T.);
#7954=EDGE_CURVE('',#6559,#6559,#726,.T.);
#7955=EDGE_CURVE('',#6559,#6560,#3764,.T.);
#7956=EDGE_CURVE('',#6560,#6560,#727,.T.);
#7957=EDGE_CURVE('',#6561,#6561,#728,.T.);
#7958=EDGE_CURVE('',#6561,#6562,#3765,.T.);
#7959=EDGE_CURVE('',#6562,#6562,#729,.T.);
#7960=EDGE_CURVE('',#6563,#6563,#730,.T.);
#7961=EDGE_CURVE('',#6563,#6564,#3766,.T.);
#7962=EDGE_CURVE('',#6564,#6564,#731,.T.);
#7963=EDGE_CURVE('',#6565,#6565,#732,.T.);
#7964=EDGE_CURVE('',#6565,#6566,#3767,.T.);
#7965=EDGE_CURVE('',#6566,#6566,#733,.T.);
#7966=EDGE_CURVE('',#6567,#6567,#734,.T.);
#7967=EDGE_CURVE('',#6567,#6568,#3768,.T.);
#7968=EDGE_CURVE('',#6568,#6568,#735,.T.);
#7969=EDGE_CURVE('',#6569,#6570,#3769,.T.);
#7970=EDGE_CURVE('',#6571,#6570,#3770,.T.);
#7971=EDGE_CURVE('',#6572,#6571,#3771,.T.);
#7972=EDGE_CURVE('',#6572,#6569,#3772,.T.);
#7973=EDGE_CURVE('',#6573,#6569,#3773,.T.);
#7974=EDGE_CURVE('',#6574,#6572,#3774,.T.);
#7975=EDGE_CURVE('',#6574,#6573,#3775,.T.);
#7976=EDGE_CURVE('',#6575,#6573,#3776,.T.);
#7977=EDGE_CURVE('',#6576,#6574,#3777,.T.);
#7978=EDGE_CURVE('',#6576,#6575,#3778,.T.);
#7979=EDGE_CURVE('',#6570,#6575,#3779,.T.);
#7980=EDGE_CURVE('',#6571,#6576,#3780,.T.);
#7981=EDGE_CURVE('',#6577,#6578,#3781,.T.);
#7982=EDGE_CURVE('',#6579,#6578,#3782,.T.);
#7983=EDGE_CURVE('',#6580,#6579,#3783,.T.);
#7984=EDGE_CURVE('',#6580,#6577,#3784,.T.);
#7985=EDGE_CURVE('',#6578,#6581,#3785,.T.);
#7986=EDGE_CURVE('',#6582,#6581,#3786,.T.);
#7987=EDGE_CURVE('',#6579,#6582,#3787,.T.);
#7988=EDGE_CURVE('',#6581,#6583,#3788,.T.);
#7989=EDGE_CURVE('',#6584,#6583,#3789,.T.);
#7990=EDGE_CURVE('',#6582,#6584,#3790,.T.);
#7991=EDGE_CURVE('',#6583,#6577,#3791,.T.);
#7992=EDGE_CURVE('',#6584,#6580,#3792,.T.);
#7993=EDGE_CURVE('',#6585,#6586,#3793,.T.);
#7994=EDGE_CURVE('',#6587,#6586,#3794,.T.);
#7995=EDGE_CURVE('',#6588,#6587,#3795,.T.);
#7996=EDGE_CURVE('',#6588,#6585,#3796,.T.);
#7997=EDGE_CURVE('',#6586,#6589,#3797,.T.);
#7998=EDGE_CURVE('',#6590,#6589,#3798,.T.);
#7999=EDGE_CURVE('',#6587,#6590,#3799,.T.);
#8000=EDGE_CURVE('',#6589,#6591,#3800,.T.);
#8001=EDGE_CURVE('',#6592,#6591,#3801,.T.);
#8002=EDGE_CURVE('',#6590,#6592,#3802,.T.);
#8003=EDGE_CURVE('',#6591,#6585,#3803,.T.);
#8004=EDGE_CURVE('',#6592,#6588,#3804,.T.);
#8005=EDGE_CURVE('',#6593,#6594,#3805,.T.);
#8006=EDGE_CURVE('',#6595,#6593,#3806,.T.);
#8007=EDGE_CURVE('',#6595,#6596,#3807,.T.);
#8008=EDGE_CURVE('',#6596,#6594,#3808,.T.);
#8009=EDGE_CURVE('',#6594,#6597,#3809,.T.);
#8010=EDGE_CURVE('',#6596,#6598,#3810,.T.);
#8011=EDGE_CURVE('',#6598,#6597,#3811,.T.);
#8012=EDGE_CURVE('',#6597,#6599,#3812,.T.);
#8013=EDGE_CURVE('',#6598,#6600,#3813,.T.);
#8014=EDGE_CURVE('',#6600,#6599,#3814,.T.);
#8015=EDGE_CURVE('',#6599,#6593,#3815,.T.);
#8016=EDGE_CURVE('',#6600,#6595,#3816,.T.);
#9907=ORIENTED_EDGE('',*,*,#7837,.F.);
#9908=ORIENTED_EDGE('',*,*,#7838,.F.);
#9909=ORIENTED_EDGE('',*,*,#7839,.T.);
#9910=ORIENTED_EDGE('',*,*,#7840,.T.);
#9911=ORIENTED_EDGE('',*,*,#7841,.F.);
#9912=ORIENTED_EDGE('',*,*,#7842,.F.);
#9913=ORIENTED_EDGE('',*,*,#7843,.T.);
#9914=ORIENTED_EDGE('',*,*,#7838,.T.);
#9915=ORIENTED_EDGE('',*,*,#7844,.F.);
#9916=ORIENTED_EDGE('',*,*,#7845,.F.);
#9917=ORIENTED_EDGE('',*,*,#7846,.T.);
#9918=ORIENTED_EDGE('',*,*,#7842,.T.);
#9919=ORIENTED_EDGE('',*,*,#7847,.F.);
#9920=ORIENTED_EDGE('',*,*,#7840,.F.);
#9921=ORIENTED_EDGE('',*,*,#7848,.T.);
#9922=ORIENTED_EDGE('',*,*,#7845,.T.);
#9923=ORIENTED_EDGE('',*,*,#7839,.F.);
#9924=ORIENTED_EDGE('',*,*,#7843,.F.);
#9925=ORIENTED_EDGE('',*,*,#7846,.F.);
#9926=ORIENTED_EDGE('',*,*,#7848,.F.);
#9927=ORIENTED_EDGE('',*,*,#7849,.T.);
#9928=ORIENTED_EDGE('',*,*,#7850,.T.);
#9929=ORIENTED_EDGE('',*,*,#7851,.T.);
#9930=ORIENTED_EDGE('',*,*,#7852,.T.);
#9931=ORIENTED_EDGE('',*,*,#7837,.T.);
#9932=ORIENTED_EDGE('',*,*,#7847,.T.);
#9933=ORIENTED_EDGE('',*,*,#7844,.T.);
#9934=ORIENTED_EDGE('',*,*,#7841,.T.);
#9935=ORIENTED_EDGE('',*,*,#7853,.F.);
#9936=ORIENTED_EDGE('',*,*,#7854,.F.);
#9937=ORIENTED_EDGE('',*,*,#7855,.F.);
#9938=ORIENTED_EDGE('',*,*,#7856,.F.);
#9939=ORIENTED_EDGE('',*,*,#7854,.T.);
#9940=ORIENTED_EDGE('',*,*,#7857,.F.);
#9941=ORIENTED_EDGE('',*,*,#7849,.F.);
#9942=ORIENTED_EDGE('',*,*,#7858,.T.);
#9943=ORIENTED_EDGE('',*,*,#7855,.T.);
#9944=ORIENTED_EDGE('',*,*,#7858,.F.);
#9945=ORIENTED_EDGE('',*,*,#7852,.F.);
#9946=ORIENTED_EDGE('',*,*,#7859,.T.);
#9947=ORIENTED_EDGE('',*,*,#7856,.T.);
#9948=ORIENTED_EDGE('',*,*,#7859,.F.);
#9949=ORIENTED_EDGE('',*,*,#7851,.F.);
#9950=ORIENTED_EDGE('',*,*,#7860,.T.);
#9951=ORIENTED_EDGE('',*,*,#7853,.T.);
#9952=ORIENTED_EDGE('',*,*,#7860,.F.);
#9953=ORIENTED_EDGE('',*,*,#7850,.F.);
#9954=ORIENTED_EDGE('',*,*,#7857,.T.);
#9955=ORIENTED_EDGE('',*,*,#7861,.T.);
#9956=ORIENTED_EDGE('',*,*,#7862,.F.);
#9957=ORIENTED_EDGE('',*,*,#7863,.F.);
#9958=ORIENTED_EDGE('',*,*,#7864,.T.);
#9959=ORIENTED_EDGE('',*,*,#7865,.T.);
#9960=ORIENTED_EDGE('',*,*,#7866,.F.);
#9961=ORIENTED_EDGE('',*,*,#7867,.F.);
#9962=ORIENTED_EDGE('',*,*,#7862,.T.);
#9963=ORIENTED_EDGE('',*,*,#7868,.T.);
#9964=ORIENTED_EDGE('',*,*,#7869,.F.);
#9965=ORIENTED_EDGE('',*,*,#7870,.F.);
#9966=ORIENTED_EDGE('',*,*,#7866,.T.);
#9967=ORIENTED_EDGE('',*,*,#7871,.T.);
#9968=ORIENTED_EDGE('',*,*,#7872,.F.);
#9969=ORIENTED_EDGE('',*,*,#7873,.F.);
#9970=ORIENTED_EDGE('',*,*,#7869,.T.);
#9971=ORIENTED_EDGE('',*,*,#7874,.T.);
#9972=ORIENTED_EDGE('',*,*,#7875,.F.);
#9973=ORIENTED_EDGE('',*,*,#7876,.F.);
#9974=ORIENTED_EDGE('',*,*,#7872,.T.);
#9975=ORIENTED_EDGE('',*,*,#7877,.T.);
#9976=ORIENTED_EDGE('',*,*,#7864,.F.);
#9977=ORIENTED_EDGE('',*,*,#7878,.F.);
#9978=ORIENTED_EDGE('',*,*,#7875,.T.);
#9979=ORIENTED_EDGE('',*,*,#7863,.T.);
#9980=ORIENTED_EDGE('',*,*,#7867,.T.);
#9981=ORIENTED_EDGE('',*,*,#7870,.T.);
#9982=ORIENTED_EDGE('',*,*,#7873,.T.);
#9983=ORIENTED_EDGE('',*,*,#7876,.T.);
#9984=ORIENTED_EDGE('',*,*,#7878,.T.);
#9985=ORIENTED_EDGE('',*,*,#7861,.F.);
#9986=ORIENTED_EDGE('',*,*,#7877,.F.);
#9987=ORIENTED_EDGE('',*,*,#7874,.F.);
#9988=ORIENTED_EDGE('',*,*,#7871,.F.);
#9989=ORIENTED_EDGE('',*,*,#7868,.F.);
#9990=ORIENTED_EDGE('',*,*,#7865,.F.);
#9991=ORIENTED_EDGE('',*,*,#7879,.F.);
#9992=ORIENTED_EDGE('',*,*,#7880,.F.);
#9993=ORIENTED_EDGE('',*,*,#7881,.T.);
#9994=ORIENTED_EDGE('',*,*,#7882,.T.);
#9995=ORIENTED_EDGE('',*,*,#7883,.F.);
#9996=ORIENTED_EDGE('',*,*,#7882,.F.);
#9997=ORIENTED_EDGE('',*,*,#7884,.T.);
#9998=ORIENTED_EDGE('',*,*,#7885,.T.);
#9999=ORIENTED_EDGE('',*,*,#7886,.F.);
#10000=ORIENTED_EDGE('',*,*,#7885,.F.);
#10001=ORIENTED_EDGE('',*,*,#7887,.T.);
#10002=ORIENTED_EDGE('',*,*,#7888,.T.);
#10003=ORIENTED_EDGE('',*,*,#7889,.F.);
#10004=ORIENTED_EDGE('',*,*,#7888,.F.);
#10005=ORIENTED_EDGE('',*,*,#7890,.T.);
#10006=ORIENTED_EDGE('',*,*,#7891,.T.);
#10007=ORIENTED_EDGE('',*,*,#7892,.F.);
#10008=ORIENTED_EDGE('',*,*,#7891,.F.);
#10009=ORIENTED_EDGE('',*,*,#7893,.T.);
#10010=ORIENTED_EDGE('',*,*,#7894,.T.);
#10011=ORIENTED_EDGE('',*,*,#7895,.F.);
#10012=ORIENTED_EDGE('',*,*,#7894,.F.);
#10013=ORIENTED_EDGE('',*,*,#7896,.T.);
#10014=ORIENTED_EDGE('',*,*,#7880,.T.);
#10015=ORIENTED_EDGE('',*,*,#7881,.F.);
#10016=ORIENTED_EDGE('',*,*,#7896,.F.);
#10017=ORIENTED_EDGE('',*,*,#7893,.F.);
#10018=ORIENTED_EDGE('',*,*,#7890,.F.);
#10019=ORIENTED_EDGE('',*,*,#7887,.F.);
#10020=ORIENTED_EDGE('',*,*,#7884,.F.);
#10021=ORIENTED_EDGE('',*,*,#7879,.T.);
#10022=ORIENTED_EDGE('',*,*,#7883,.T.);
#10023=ORIENTED_EDGE('',*,*,#7886,.T.);
#10024=ORIENTED_EDGE('',*,*,#7889,.T.);
#10025=ORIENTED_EDGE('',*,*,#7892,.T.);
#10026=ORIENTED_EDGE('',*,*,#7895,.T.);
#10027=ORIENTED_EDGE('',*,*,#7897,.T.);
#10028=ORIENTED_EDGE('',*,*,#7898,.T.);
#10029=ORIENTED_EDGE('',*,*,#7899,.F.);
#10030=ORIENTED_EDGE('',*,*,#7898,.F.);
#10031=ORIENTED_EDGE('',*,*,#7900,.T.);
#10032=ORIENTED_EDGE('',*,*,#7901,.T.);
#10033=ORIENTED_EDGE('',*,*,#7902,.F.);
#10034=ORIENTED_EDGE('',*,*,#7901,.F.);
#10035=ORIENTED_EDGE('',*,*,#7903,.T.);
#10036=ORIENTED_EDGE('',*,*,#7904,.T.);
#10037=ORIENTED_EDGE('',*,*,#7905,.F.);
#10038=ORIENTED_EDGE('',*,*,#7904,.F.);
#10039=ORIENTED_EDGE('',*,*,#7906,.T.);
#10040=ORIENTED_EDGE('',*,*,#7907,.T.);
#10041=ORIENTED_EDGE('',*,*,#7908,.F.);
#10042=ORIENTED_EDGE('',*,*,#7907,.F.);
#10043=ORIENTED_EDGE('',*,*,#7909,.T.);
#10044=ORIENTED_EDGE('',*,*,#7910,.T.);
#10045=ORIENTED_EDGE('',*,*,#7911,.F.);
#10046=ORIENTED_EDGE('',*,*,#7910,.F.);
#10047=ORIENTED_EDGE('',*,*,#7912,.T.);
#10048=ORIENTED_EDGE('',*,*,#7913,.T.);
#10049=ORIENTED_EDGE('',*,*,#7914,.F.);
#10050=ORIENTED_EDGE('',*,*,#7913,.F.);
#10051=ORIENTED_EDGE('',*,*,#7915,.T.);
#10052=ORIENTED_EDGE('',*,*,#7916,.T.);
#10053=ORIENTED_EDGE('',*,*,#7917,.T.);
#10054=ORIENTED_EDGE('',*,*,#7918,.T.);
#10055=ORIENTED_EDGE('',*,*,#7909,.F.);
#10056=ORIENTED_EDGE('',*,*,#7903,.F.);
#10057=ORIENTED_EDGE('',*,*,#7897,.F.);
#10058=ORIENTED_EDGE('',*,*,#7900,.F.);
#10059=ORIENTED_EDGE('',*,*,#7906,.F.);
#10060=ORIENTED_EDGE('',*,*,#7912,.F.);
#10061=ORIENTED_EDGE('',*,*,#7919,.F.);
#10062=ORIENTED_EDGE('',*,*,#7920,.F.);
#10063=ORIENTED_EDGE('',*,*,#7921,.F.);
#10064=ORIENTED_EDGE('',*,*,#7922,.F.);
#10065=ORIENTED_EDGE('',*,*,#7914,.T.);
#10066=ORIENTED_EDGE('',*,*,#7911,.T.);
#10067=ORIENTED_EDGE('',*,*,#7908,.T.);
#10068=ORIENTED_EDGE('',*,*,#7905,.T.);
#10069=ORIENTED_EDGE('',*,*,#7902,.T.);
#10070=ORIENTED_EDGE('',*,*,#7899,.T.);
#10071=ORIENTED_EDGE('',*,*,#7919,.T.);
#10072=ORIENTED_EDGE('',*,*,#7923,.F.);
#10073=ORIENTED_EDGE('',*,*,#7915,.F.);
#10074=ORIENTED_EDGE('',*,*,#7924,.T.);
#10075=ORIENTED_EDGE('',*,*,#7922,.T.);
#10076=ORIENTED_EDGE('',*,*,#7925,.F.);
#10077=ORIENTED_EDGE('',*,*,#7916,.F.);
#10078=ORIENTED_EDGE('',*,*,#7923,.T.);
#10079=ORIENTED_EDGE('',*,*,#7921,.T.);
#10080=ORIENTED_EDGE('',*,*,#7926,.F.);
#10081=ORIENTED_EDGE('',*,*,#7917,.F.);
#10082=ORIENTED_EDGE('',*,*,#7925,.T.);
#10083=ORIENTED_EDGE('',*,*,#7920,.T.);
#10084=ORIENTED_EDGE('',*,*,#7924,.F.);
#10085=ORIENTED_EDGE('',*,*,#7918,.F.);
#10086=ORIENTED_EDGE('',*,*,#7926,.T.);
#10087=ORIENTED_EDGE('',*,*,#7927,.F.);
#10088=ORIENTED_EDGE('',*,*,#7928,.T.);
#10089=ORIENTED_EDGE('',*,*,#7929,.T.);
#10090=ORIENTED_EDGE('',*,*,#7928,.F.);
#10091=ORIENTED_EDGE('',*,*,#7930,.F.);
#10092=ORIENTED_EDGE('',*,*,#7931,.T.);
#10093=ORIENTED_EDGE('',*,*,#7932,.T.);
#10094=ORIENTED_EDGE('',*,*,#7931,.F.);
#10095=ORIENTED_EDGE('',*,*,#7933,.F.);
#10096=ORIENTED_EDGE('',*,*,#7934,.T.);
#10097=ORIENTED_EDGE('',*,*,#7935,.T.);
#10098=ORIENTED_EDGE('',*,*,#7934,.F.);
#10099=ORIENTED_EDGE('',*,*,#7936,.F.);
#10100=ORIENTED_EDGE('',*,*,#7937,.T.);
#10101=ORIENTED_EDGE('',*,*,#7938,.T.);
#10102=ORIENTED_EDGE('',*,*,#7937,.F.);
#10103=ORIENTED_EDGE('',*,*,#7939,.F.);
#10104=ORIENTED_EDGE('',*,*,#7940,.T.);
#10105=ORIENTED_EDGE('',*,*,#7941,.T.);
#10106=ORIENTED_EDGE('',*,*,#7940,.F.);
#10107=ORIENTED_EDGE('',*,*,#7942,.F.);
#10108=ORIENTED_EDGE('',*,*,#7943,.F.);
#10109=ORIENTED_EDGE('',*,*,#7944,.T.);
#10110=ORIENTED_EDGE('',*,*,#7945,.T.);
#10111=ORIENTED_EDGE('',*,*,#7946,.F.);
#10112=ORIENTED_EDGE('',*,*,#7947,.F.);
#10113=ORIENTED_EDGE('',*,*,#7948,.T.);
#10114=ORIENTED_EDGE('',*,*,#7943,.T.);
#10115=ORIENTED_EDGE('',*,*,#7949,.F.);
#10116=ORIENTED_EDGE('',*,*,#7950,.F.);
#10117=ORIENTED_EDGE('',*,*,#7951,.T.);
#10118=ORIENTED_EDGE('',*,*,#7947,.T.);
#10119=ORIENTED_EDGE('',*,*,#7952,.F.);
#10120=ORIENTED_EDGE('',*,*,#7945,.F.);
#10121=ORIENTED_EDGE('',*,*,#7953,.T.);
#10122=ORIENTED_EDGE('',*,*,#7950,.T.);
#10123=ORIENTED_EDGE('',*,*,#7944,.F.);
#10124=ORIENTED_EDGE('',*,*,#7948,.F.);
#10125=ORIENTED_EDGE('',*,*,#7951,.F.);
#10126=ORIENTED_EDGE('',*,*,#7953,.F.);
#10127=ORIENTED_EDGE('',*,*,#7927,.T.);
#10128=ORIENTED_EDGE('',*,*,#7930,.T.);
#10129=ORIENTED_EDGE('',*,*,#7933,.T.);
#10130=ORIENTED_EDGE('',*,*,#7936,.T.);
#10131=ORIENTED_EDGE('',*,*,#7939,.T.);
#10132=ORIENTED_EDGE('',*,*,#7942,.T.);
#10133=ORIENTED_EDGE('',*,*,#7952,.T.);
#10134=ORIENTED_EDGE('',*,*,#7949,.T.);
#10135=ORIENTED_EDGE('',*,*,#7946,.T.);
#10136=ORIENTED_EDGE('',*,*,#7929,.F.);
#10137=ORIENTED_EDGE('',*,*,#7932,.F.);
#10138=ORIENTED_EDGE('',*,*,#7935,.F.);
#10139=ORIENTED_EDGE('',*,*,#7938,.F.);
#10140=ORIENTED_EDGE('',*,*,#7941,.F.);
#10141=ORIENTED_EDGE('',*,*,#7954,.T.);
#10142=ORIENTED_EDGE('',*,*,#7955,.T.);
#10143=ORIENTED_EDGE('',*,*,#7956,.F.);
#10144=ORIENTED_EDGE('',*,*,#7955,.F.);
#10145=ORIENTED_EDGE('',*,*,#7957,.T.);
#10146=ORIENTED_EDGE('',*,*,#7958,.T.);
#10147=ORIENTED_EDGE('',*,*,#7959,.F.);
#10148=ORIENTED_EDGE('',*,*,#7958,.F.);
#10149=ORIENTED_EDGE('',*,*,#7960,.T.);
#10150=ORIENTED_EDGE('',*,*,#7961,.T.);
#10151=ORIENTED_EDGE('',*,*,#7962,.F.);
#10152=ORIENTED_EDGE('',*,*,#7961,.F.);
#10153=ORIENTED_EDGE('',*,*,#7963,.T.);
#10154=ORIENTED_EDGE('',*,*,#7964,.T.);
#10155=ORIENTED_EDGE('',*,*,#7965,.F.);
#10156=ORIENTED_EDGE('',*,*,#7964,.F.);
#10157=ORIENTED_EDGE('',*,*,#7966,.T.);
#10158=ORIENTED_EDGE('',*,*,#7967,.T.);
#10159=ORIENTED_EDGE('',*,*,#7968,.F.);
#10160=ORIENTED_EDGE('',*,*,#7967,.F.);
#10161=ORIENTED_EDGE('',*,*,#7969,.T.);
#10162=ORIENTED_EDGE('',*,*,#7970,.F.);
#10163=ORIENTED_EDGE('',*,*,#7971,.F.);
#10164=ORIENTED_EDGE('',*,*,#7972,.T.);
#10165=ORIENTED_EDGE('',*,*,#7973,.T.);
#10166=ORIENTED_EDGE('',*,*,#7972,.F.);
#10167=ORIENTED_EDGE('',*,*,#7974,.F.);
#10168=ORIENTED_EDGE('',*,*,#7975,.T.);
#10169=ORIENTED_EDGE('',*,*,#7976,.T.);
#10170=ORIENTED_EDGE('',*,*,#7975,.F.);
#10171=ORIENTED_EDGE('',*,*,#7977,.F.);
#10172=ORIENTED_EDGE('',*,*,#7978,.T.);
#10173=ORIENTED_EDGE('',*,*,#7979,.T.);
#10174=ORIENTED_EDGE('',*,*,#7978,.F.);
#10175=ORIENTED_EDGE('',*,*,#7980,.F.);
#10176=ORIENTED_EDGE('',*,*,#7970,.T.);
#10177=ORIENTED_EDGE('',*,*,#7971,.T.);
#10178=ORIENTED_EDGE('',*,*,#7980,.T.);
#10179=ORIENTED_EDGE('',*,*,#7977,.T.);
#10180=ORIENTED_EDGE('',*,*,#7974,.T.);
#10181=ORIENTED_EDGE('',*,*,#7954,.F.);
#10182=ORIENTED_EDGE('',*,*,#7957,.F.);
#10183=ORIENTED_EDGE('',*,*,#7960,.F.);
#10184=ORIENTED_EDGE('',*,*,#7963,.F.);
#10185=ORIENTED_EDGE('',*,*,#7966,.F.);
#10186=ORIENTED_EDGE('',*,*,#7969,.F.);
#10187=ORIENTED_EDGE('',*,*,#7973,.F.);
#10188=ORIENTED_EDGE('',*,*,#7976,.F.);
#10189=ORIENTED_EDGE('',*,*,#7979,.F.);
#10190=ORIENTED_EDGE('',*,*,#7956,.T.);
#10191=ORIENTED_EDGE('',*,*,#7959,.T.);
#10192=ORIENTED_EDGE('',*,*,#7962,.T.);
#10193=ORIENTED_EDGE('',*,*,#7965,.T.);
#10194=ORIENTED_EDGE('',*,*,#7968,.T.);
#10195=ORIENTED_EDGE('',*,*,#7981,.T.);
#10196=ORIENTED_EDGE('',*,*,#7982,.F.);
#10197=ORIENTED_EDGE('',*,*,#7983,.F.);
#10198=ORIENTED_EDGE('',*,*,#7984,.T.);
#10199=ORIENTED_EDGE('',*,*,#7985,.T.);
#10200=ORIENTED_EDGE('',*,*,#7986,.F.);
#10201=ORIENTED_EDGE('',*,*,#7987,.F.);
#10202=ORIENTED_EDGE('',*,*,#7982,.T.);
#10203=ORIENTED_EDGE('',*,*,#7988,.T.);
#10204=ORIENTED_EDGE('',*,*,#7989,.F.);
#10205=ORIENTED_EDGE('',*,*,#7990,.F.);
#10206=ORIENTED_EDGE('',*,*,#7986,.T.);
#10207=ORIENTED_EDGE('',*,*,#7991,.T.);
#10208=ORIENTED_EDGE('',*,*,#7984,.F.);
#10209=ORIENTED_EDGE('',*,*,#7992,.F.);
#10210=ORIENTED_EDGE('',*,*,#7989,.T.);
#10211=ORIENTED_EDGE('',*,*,#7983,.T.);
#10212=ORIENTED_EDGE('',*,*,#7987,.T.);
#10213=ORIENTED_EDGE('',*,*,#7990,.T.);
#10214=ORIENTED_EDGE('',*,*,#7992,.T.);
#10215=ORIENTED_EDGE('',*,*,#7981,.F.);
#10216=ORIENTED_EDGE('',*,*,#7991,.F.);
#10217=ORIENTED_EDGE('',*,*,#7988,.F.);
#10218=ORIENTED_EDGE('',*,*,#7985,.F.);
#10219=ORIENTED_EDGE('',*,*,#7993,.T.);
#10220=ORIENTED_EDGE('',*,*,#7994,.F.);
#10221=ORIENTED_EDGE('',*,*,#7995,.F.);
#10222=ORIENTED_EDGE('',*,*,#7996,.T.);
#10223=ORIENTED_EDGE('',*,*,#7997,.T.);
#10224=ORIENTED_EDGE('',*,*,#7998,.F.);
#10225=ORIENTED_EDGE('',*,*,#7999,.F.);
#10226=ORIENTED_EDGE('',*,*,#7994,.T.);
#10227=ORIENTED_EDGE('',*,*,#8000,.T.);
#10228=ORIENTED_EDGE('',*,*,#8001,.F.);
#10229=ORIENTED_EDGE('',*,*,#8002,.F.);
#10230=ORIENTED_EDGE('',*,*,#7998,.T.);
#10231=ORIENTED_EDGE('',*,*,#8003,.T.);
#10232=ORIENTED_EDGE('',*,*,#7996,.F.);
#10233=ORIENTED_EDGE('',*,*,#8004,.F.);
#10234=ORIENTED_EDGE('',*,*,#8001,.T.);
#10235=ORIENTED_EDGE('',*,*,#7995,.T.);
#10236=ORIENTED_EDGE('',*,*,#7999,.T.);
#10237=ORIENTED_EDGE('',*,*,#8002,.T.);
#10238=ORIENTED_EDGE('',*,*,#8004,.T.);
#10239=ORIENTED_EDGE('',*,*,#7993,.F.);
#10240=ORIENTED_EDGE('',*,*,#8003,.F.);
#10241=ORIENTED_EDGE('',*,*,#8000,.F.);
#10242=ORIENTED_EDGE('',*,*,#7997,.F.);
#10243=ORIENTED_EDGE('',*,*,#8005,.F.);
#10244=ORIENTED_EDGE('',*,*,#8006,.F.);
#10245=ORIENTED_EDGE('',*,*,#8007,.T.);
#10246=ORIENTED_EDGE('',*,*,#8008,.T.);
#10247=ORIENTED_EDGE('',*,*,#8009,.F.);
#10248=ORIENTED_EDGE('',*,*,#8008,.F.);
#10249=ORIENTED_EDGE('',*,*,#8010,.T.);
#10250=ORIENTED_EDGE('',*,*,#8011,.T.);
#10251=ORIENTED_EDGE('',*,*,#8012,.F.);
#10252=ORIENTED_EDGE('',*,*,#8011,.F.);
#10253=ORIENTED_EDGE('',*,*,#8013,.T.);
#10254=ORIENTED_EDGE('',*,*,#8014,.T.);
#10255=ORIENTED_EDGE('',*,*,#8015,.F.);
#10256=ORIENTED_EDGE('',*,*,#8014,.F.);
#10257=ORIENTED_EDGE('',*,*,#8016,.T.);
#10258=ORIENTED_EDGE('',*,*,#8006,.T.);
#10259=ORIENTED_EDGE('',*,*,#8007,.F.);
#10260=ORIENTED_EDGE('',*,*,#8016,.F.);
#10261=ORIENTED_EDGE('',*,*,#8013,.F.);
#10262=ORIENTED_EDGE('',*,*,#8010,.F.);
#10263=ORIENTED_EDGE('',*,*,#8005,.T.);
#10264=ORIENTED_EDGE('',*,*,#8009,.T.);
#10265=ORIENTED_EDGE('',*,*,#8012,.T.);
#10266=ORIENTED_EDGE('',*,*,#8015,.T.);
#14047=PLANE('',#15785);
#14048=PLANE('',#15786);
#14049=PLANE('',#15787);
#14050=PLANE('',#15788);
#14051=PLANE('',#15789);
#14052=PLANE('',#15790);
#14053=PLANE('',#15791);
#14054=PLANE('',#15792);
#14055=PLANE('',#15793);
#14056=PLANE('',#15794);
#14057=PLANE('',#15795);
#14058=PLANE('',#15796);
#14059=PLANE('',#15800);
#14060=PLANE('',#15801);
#14061=PLANE('',#15802);
#14062=PLANE('',#15803);
#14063=PLANE('',#15804);
#14064=PLANE('',#15805);
#14065=PLANE('',#15806);
#14066=PLANE('',#15810);
#14067=PLANE('',#15811);
#14068=PLANE('',#15812);
#14069=PLANE('',#15813);
#14070=PLANE('',#15814);
#14071=PLANE('',#15833);
#14072=PLANE('',#15834);
#14073=PLANE('',#15835);
#14074=PLANE('',#15836);
#14075=PLANE('',#15837);
#14076=PLANE('',#15838);
#14077=PLANE('',#15854);
#14078=PLANE('',#15855);
#14079=PLANE('',#15856);
#14080=PLANE('',#15857);
#14081=PLANE('',#15858);
#14082=PLANE('',#15859);
#14083=PLANE('',#15875);
#14084=PLANE('',#15876);
#14085=PLANE('',#15877);
#14086=PLANE('',#15878);
#14087=PLANE('',#15879);
#14088=PLANE('',#15880);
#14089=PLANE('',#15881);
#14090=PLANE('',#15882);
#14091=PLANE('',#15883);
#14092=PLANE('',#15884);
#14093=PLANE('',#15885);
#14094=PLANE('',#15886);
#14095=PLANE('',#15887);
#14096=PLANE('',#15888);
#14097=PLANE('',#15889);
#14098=PLANE('',#15890);
#14099=PLANE('',#15891);
#14100=PLANE('',#15892);
#14101=PLANE('',#15893);
#14102=PLANE('',#15894);
#14103=PLANE('',#15895);
#14104=PLANE('',#15896);
#14105=PLANE('',#15897);
#14106=PLANE('',#15898);
#14644=ADVANCED_FACE('',(#1676),#14047,.T.);
#14645=ADVANCED_FACE('',(#1677),#14048,.T.);
#14646=ADVANCED_FACE('',(#1678),#14049,.T.);
#14647=ADVANCED_FACE('',(#1679),#14050,.T.);
#14648=ADVANCED_FACE('',(#1680,#1469),#14051,.T.);
#14649=ADVANCED_FACE('',(#1681,#1470),#14052,.F.);
#14650=ADVANCED_FACE('',(#1682),#14053,.F.);
#14651=ADVANCED_FACE('',(#1683),#14054,.F.);
#14652=ADVANCED_FACE('',(#1684),#14055,.F.);
#14653=ADVANCED_FACE('',(#1685),#14056,.F.);
#14654=ADVANCED_FACE('',(#1686),#14057,.F.);
#14655=ADVANCED_FACE('',(#1687),#14058,.F.);
#14656=ADVANCED_FACE('',(#1688),#1081,.F.);
#14657=ADVANCED_FACE('',(#1689),#14059,.F.);
#14658=ADVANCED_FACE('',(#1690),#14060,.F.);
#14659=ADVANCED_FACE('',(#1691),#14061,.F.);
#14660=ADVANCED_FACE('',(#1692),#14062,.T.);
#14661=ADVANCED_FACE('',(#1693),#14063,.F.);
#14662=ADVANCED_FACE('',(#1694),#14064,.F.);
#14663=ADVANCED_FACE('',(#1695),#14065,.F.);
#14664=ADVANCED_FACE('',(#1696),#1082,.F.);
#14665=ADVANCED_FACE('',(#1697),#14066,.F.);
#14666=ADVANCED_FACE('',(#1698),#14067,.F.);
#14667=ADVANCED_FACE('',(#1699),#14068,.F.);
#14668=ADVANCED_FACE('',(#1700),#14069,.T.);
#14669=ADVANCED_FACE('',(#1701),#14070,.F.);
#14670=ADVANCED_FACE('',(#1702),#1083,.F.);
#14671=ADVANCED_FACE('',(#1703),#1084,.F.);
#14672=ADVANCED_FACE('',(#1704),#1085,.F.);
#14673=ADVANCED_FACE('',(#1705),#1086,.F.);
#14674=ADVANCED_FACE('',(#1706),#1087,.F.);
#14675=ADVANCED_FACE('',(#1707),#1088,.F.);
#14676=ADVANCED_FACE('',(#1708,#1471,#1472,#1473,#1474,#1475,#1476),#14071,
 .T.);
#14677=ADVANCED_FACE('',(#1709,#1477,#1478,#1479,#1480,#1481,#1482),#14072,
 .F.);
#14678=ADVANCED_FACE('',(#1710),#14073,.F.);
#14679=ADVANCED_FACE('',(#1711),#14074,.F.);
#14680=ADVANCED_FACE('',(#1712),#14075,.F.);
#14681=ADVANCED_FACE('',(#1713),#14076,.F.);
#14682=ADVANCED_FACE('',(#1714),#1089,.F.);
#14683=ADVANCED_FACE('',(#1715),#1090,.F.);
#14684=ADVANCED_FACE('',(#1716),#1091,.F.);
#14685=ADVANCED_FACE('',(#1717),#1092,.F.);
#14686=ADVANCED_FACE('',(#1718),#1093,.F.);
#14687=ADVANCED_FACE('',(#1719),#14077,.T.);
#14688=ADVANCED_FACE('',(#1720),#14078,.T.);
#14689=ADVANCED_FACE('',(#1721),#14079,.T.);
#14690=ADVANCED_FACE('',(#1722),#14080,.T.);
#14691=ADVANCED_FACE('',(#1723,#1483,#1484,#1485,#1486,#1487),#14081,.T.);
#14692=ADVANCED_FACE('',(#1724,#1488,#1489,#1490,#1491,#1492),#14082,.F.);
#14693=ADVANCED_FACE('',(#1725),#1094,.F.);
#14694=ADVANCED_FACE('',(#1726),#1095,.F.);
#14695=ADVANCED_FACE('',(#1727),#1096,.F.);
#14696=ADVANCED_FACE('',(#1728),#1097,.F.);
#14697=ADVANCED_FACE('',(#1729),#1098,.F.);
#14698=ADVANCED_FACE('',(#1730),#14083,.T.);
#14699=ADVANCED_FACE('',(#1731),#14084,.T.);
#14700=ADVANCED_FACE('',(#1732),#14085,.T.);
#14701=ADVANCED_FACE('',(#1733),#14086,.T.);
#14702=ADVANCED_FACE('',(#1734,#1493,#1494,#1495,#1496,#1497),#14087,.T.);
#14703=ADVANCED_FACE('',(#1735,#1498,#1499,#1500,#1501,#1502),#14088,.F.);
#14704=ADVANCED_FACE('',(#1736),#14089,.F.);
#14705=ADVANCED_FACE('',(#1737),#14090,.F.);
#14706=ADVANCED_FACE('',(#1738),#14091,.F.);
#14707=ADVANCED_FACE('',(#1739),#14092,.F.);
#14708=ADVANCED_FACE('',(#1740),#14093,.T.);
#14709=ADVANCED_FACE('',(#1741),#14094,.F.);
#14710=ADVANCED_FACE('',(#1742),#14095,.F.);
#14711=ADVANCED_FACE('',(#1743),#14096,.F.);
#14712=ADVANCED_FACE('',(#1744),#14097,.F.);
#14713=ADVANCED_FACE('',(#1745),#14098,.F.);
#14714=ADVANCED_FACE('',(#1746),#14099,.F.);
#14715=ADVANCED_FACE('',(#1747),#14100,.T.);
#14716=ADVANCED_FACE('',(#1748),#14101,.F.);
#14717=ADVANCED_FACE('',(#1749),#14102,.F.);
#14718=ADVANCED_FACE('',(#1750),#14103,.F.);
#14719=ADVANCED_FACE('',(#1751),#14104,.F.);
#14720=ADVANCED_FACE('',(#1752),#14105,.F.);
#14721=ADVANCED_FACE('',(#1753),#14106,.T.);
#15539=CLOSED_SHELL('',(#14644,#14645,#14646,#14647,#14648,#14649,#14650,
#14651,#14652,#14653));
#15540=CLOSED_SHELL('',(#14654,#14655,#14656,#14657,#14658,#14659,#14660,
#14661));
#15541=CLOSED_SHELL('',(#14662,#14663,#14664,#14665,#14666,#14667,#14668,
#14669));
#15542=CLOSED_SHELL('',(#14670,#14671,#14672,#14673,#14674,#14675,#14676,
#14677,#14678,#14679,#14680,#14681));
#15543=CLOSED_SHELL('',(#14682,#14683,#14684,#14685,#14686,#14687,#14688,
#14689,#14690,#14691,#14692));
#15544=CLOSED_SHELL('',(#14693,#14694,#14695,#14696,#14697,#14698,#14699,
#14700,#14701,#14702,#14703));
#15545=CLOSED_SHELL('',(#14704,#14705,#14706,#14707,#14708,#14709));
#15546=CLOSED_SHELL('',(#14710,#14711,#14712,#14713,#14714,#14715));
#15547=CLOSED_SHELL('',(#14716,#14717,#14718,#14719,#14720,#14721));
#15784=AXIS2_PLACEMENT_3D('',#21310,#17159,#17160);
#15785=AXIS2_PLACEMENT_3D('',#21311,#17161,#17162);
#15786=AXIS2_PLACEMENT_3D('',#21320,#17167,#17168);
#15787=AXIS2_PLACEMENT_3D('',#21326,#17172,#17173);
#15788=AXIS2_PLACEMENT_3D('',#21332,#17177,#17178);
#15789=AXIS2_PLACEMENT_3D('',#21335,#17181,#17182);
#15790=AXIS2_PLACEMENT_3D('',#21344,#17187,#17188);
#15791=AXIS2_PLACEMENT_3D('',#21353,#17193,#17194);
#15792=AXIS2_PLACEMENT_3D('',#21356,#17197,#17198);
#15793=AXIS2_PLACEMENT_3D('',#21358,#17200,#17201);
#15794=AXIS2_PLACEMENT_3D('',#21360,#17203,#17204);
#15795=AXIS2_PLACEMENT_3D('',#21361,#17205,#17206);
#15796=AXIS2_PLACEMENT_3D('',#21370,#17211,#17212);
#15797=AXIS2_PLACEMENT_3D('',#21376,#17216,#17217);
#15798=AXIS2_PLACEMENT_3D('',#21378,#17218,#17219);
#15799=AXIS2_PLACEMENT_3D('',#21381,#17221,#17222);
#15800=AXIS2_PLACEMENT_3D('',#21382,#17223,#17224);
#15801=AXIS2_PLACEMENT_3D('',#21388,#17228,#17229);
#15802=AXIS2_PLACEMENT_3D('',#21394,#17233,#17234);
#15803=AXIS2_PLACEMENT_3D('',#21397,#17237,#17238);
#15804=AXIS2_PLACEMENT_3D('',#21398,#17239,#17240);
#15805=AXIS2_PLACEMENT_3D('',#21399,#17241,#17242);
#15806=AXIS2_PLACEMENT_3D('',#21408,#17247,#17248);
#15807=AXIS2_PLACEMENT_3D('',#21414,#17252,#17253);
#15808=AXIS2_PLACEMENT_3D('',#21416,#17254,#17255);
#15809=AXIS2_PLACEMENT_3D('',#21418,#17256,#17257);
#15810=AXIS2_PLACEMENT_3D('',#21420,#17259,#17260);
#15811=AXIS2_PLACEMENT_3D('',#21426,#17264,#17265);
#15812=AXIS2_PLACEMENT_3D('',#21432,#17269,#17270);
#15813=AXIS2_PLACEMENT_3D('',#21435,#17273,#17274);
#15814=AXIS2_PLACEMENT_3D('',#21436,#17275,#17276);
#15815=AXIS2_PLACEMENT_3D('',#21437,#17277,#17278);
#15816=AXIS2_PLACEMENT_3D('',#21439,#17279,#17280);
#15817=AXIS2_PLACEMENT_3D('',#21442,#17282,#17283);
#15818=AXIS2_PLACEMENT_3D('',#21443,#17284,#17285);
#15819=AXIS2_PLACEMENT_3D('',#21445,#17286,#17287);
#15820=AXIS2_PLACEMENT_3D('',#21448,#17289,#17290);
#15821=AXIS2_PLACEMENT_3D('',#21449,#17291,#17292);
#15822=AXIS2_PLACEMENT_3D('',#21451,#17293,#17294);
#15823=AXIS2_PLACEMENT_3D('',#21454,#17296,#17297);
#15824=AXIS2_PLACEMENT_3D('',#21455,#17298,#17299);
#15825=AXIS2_PLACEMENT_3D('',#21457,#17300,#17301);
#15826=AXIS2_PLACEMENT_3D('',#21460,#17303,#17304);
#15827=AXIS2_PLACEMENT_3D('',#21461,#17305,#17306);
#15828=AXIS2_PLACEMENT_3D('',#21463,#17307,#17308);
#15829=AXIS2_PLACEMENT_3D('',#21466,#17310,#17311);
#15830=AXIS2_PLACEMENT_3D('',#21467,#17312,#17313);
#15831=AXIS2_PLACEMENT_3D('',#21469,#17314,#17315);
#15832=AXIS2_PLACEMENT_3D('',#21472,#17317,#17318);
#15833=AXIS2_PLACEMENT_3D('',#21473,#17319,#17320);
#15834=AXIS2_PLACEMENT_3D('',#21482,#17325,#17326);
#15835=AXIS2_PLACEMENT_3D('',#21491,#17331,#17332);
#15836=AXIS2_PLACEMENT_3D('',#21494,#17335,#17336);
#15837=AXIS2_PLACEMENT_3D('',#21496,#17338,#17339);
#15838=AXIS2_PLACEMENT_3D('',#21498,#17341,#17342);
#15839=AXIS2_PLACEMENT_3D('',#21499,#17343,#17344);
#15840=AXIS2_PLACEMENT_3D('',#21501,#17345,#17346);
#15841=AXIS2_PLACEMENT_3D('',#21504,#17348,#17349);
#15842=AXIS2_PLACEMENT_3D('',#21505,#17350,#17351);
#15843=AXIS2_PLACEMENT_3D('',#21507,#17352,#17353);
#15844=AXIS2_PLACEMENT_3D('',#21510,#17355,#17356);
#15845=AXIS2_PLACEMENT_3D('',#21511,#17357,#17358);
#15846=AXIS2_PLACEMENT_3D('',#21513,#17359,#17360);
#15847=AXIS2_PLACEMENT_3D('',#21516,#17362,#17363);
#15848=AXIS2_PLACEMENT_3D('',#21517,#17364,#17365);
#15849=AXIS2_PLACEMENT_3D('',#21519,#17366,#17367);
#15850=AXIS2_PLACEMENT_3D('',#21522,#17369,#17370);
#15851=AXIS2_PLACEMENT_3D('',#21523,#17371,#17372);
#15852=AXIS2_PLACEMENT_3D('',#21525,#17373,#17374);
#15853=AXIS2_PLACEMENT_3D('',#21528,#17376,#17377);
#15854=AXIS2_PLACEMENT_3D('',#21529,#17378,#17379);
#15855=AXIS2_PLACEMENT_3D('',#21538,#17384,#17385);
#15856=AXIS2_PLACEMENT_3D('',#21544,#17389,#17390);
#15857=AXIS2_PLACEMENT_3D('',#21550,#17394,#17395);
#15858=AXIS2_PLACEMENT_3D('',#21553,#17398,#17399);
#15859=AXIS2_PLACEMENT_3D('',#21554,#17400,#17401);
#15860=AXIS2_PLACEMENT_3D('',#21555,#17402,#17403);
#15861=AXIS2_PLACEMENT_3D('',#21557,#17404,#17405);
#15862=AXIS2_PLACEMENT_3D('',#21560,#17407,#17408);
#15863=AXIS2_PLACEMENT_3D('',#21561,#17409,#17410);
#15864=AXIS2_PLACEMENT_3D('',#21563,#17411,#17412);
#15865=AXIS2_PLACEMENT_3D('',#21566,#17414,#17415);
#15866=AXIS2_PLACEMENT_3D('',#21567,#17416,#17417);
#15867=AXIS2_PLACEMENT_3D('',#21569,#17418,#17419);
#15868=AXIS2_PLACEMENT_3D('',#21572,#17421,#17422);
#15869=AXIS2_PLACEMENT_3D('',#21573,#17423,#17424);
#15870=AXIS2_PLACEMENT_3D('',#21575,#17425,#17426);
#15871=AXIS2_PLACEMENT_3D('',#21578,#17428,#17429);
#15872=AXIS2_PLACEMENT_3D('',#21579,#17430,#17431);
#15873=AXIS2_PLACEMENT_3D('',#21581,#17432,#17433);
#15874=AXIS2_PLACEMENT_3D('',#21584,#17435,#17436);
#15875=AXIS2_PLACEMENT_3D('',#21585,#17437,#17438);
#15876=AXIS2_PLACEMENT_3D('',#21594,#17443,#17444);
#15877=AXIS2_PLACEMENT_3D('',#21600,#17448,#17449);
#15878=AXIS2_PLACEMENT_3D('',#21606,#17453,#17454);
#15879=AXIS2_PLACEMENT_3D('',#21609,#17457,#17458);
#15880=AXIS2_PLACEMENT_3D('',#21610,#17459,#17460);
#15881=AXIS2_PLACEMENT_3D('',#21611,#17461,#17462);
#15882=AXIS2_PLACEMENT_3D('',#21620,#17467,#17468);
#15883=AXIS2_PLACEMENT_3D('',#21626,#17472,#17473);
#15884=AXIS2_PLACEMENT_3D('',#21632,#17477,#17478);
#15885=AXIS2_PLACEMENT_3D('',#21635,#17481,#17482);
#15886=AXIS2_PLACEMENT_3D('',#21636,#17483,#17484);
#15887=AXIS2_PLACEMENT_3D('',#21637,#17485,#17486);
#15888=AXIS2_PLACEMENT_3D('',#21646,#17491,#17492);
#15889=AXIS2_PLACEMENT_3D('',#21652,#17496,#17497);
#15890=AXIS2_PLACEMENT_3D('',#21658,#17501,#17502);
#15891=AXIS2_PLACEMENT_3D('',#21661,#17505,#17506);
#15892=AXIS2_PLACEMENT_3D('',#21662,#17507,#17508);
#15893=AXIS2_PLACEMENT_3D('',#21663,#17509,#17510);
#15894=AXIS2_PLACEMENT_3D('',#21672,#17515,#17516);
#15895=AXIS2_PLACEMENT_3D('',#21678,#17520,#17521);
#15896=AXIS2_PLACEMENT_3D('',#21684,#17525,#17526);
#15897=AXIS2_PLACEMENT_3D('',#21687,#17529,#17530);
#15898=AXIS2_PLACEMENT_3D('',#21688,#17531,#17532);
#17159=DIRECTION('axis',(0.,0.,1.));
#17160=DIRECTION('refdir',(1.,0.,0.));
#17161=DIRECTION('center_axis',(1.,0.,0.));
#17162=DIRECTION('ref_axis',(0.,0.,-1.));
#17163=DIRECTION('',(0.,1.,0.));
#17164=DIRECTION('',(0.,0.,1.));
#17165=DIRECTION('',(0.,1.,0.));
#17166=DIRECTION('',(0.,0.,1.));
#17167=DIRECTION('center_axis',(0.,-1.,0.));
#17168=DIRECTION('ref_axis',(0.,0.,-1.));
#17169=DIRECTION('',(1.,0.,0.));
#17170=DIRECTION('',(0.,0.,1.));
#17171=DIRECTION('',(1.,0.,0.));
#17172=DIRECTION('center_axis',(-1.,0.,0.));
#17173=DIRECTION('ref_axis',(0.,0.,1.));
#17174=DIRECTION('',(0.,-1.,0.));
#17175=DIRECTION('',(0.,0.,1.));
#17176=DIRECTION('',(0.,-1.,0.));
#17177=DIRECTION('center_axis',(0.,1.,0.));
#17178=DIRECTION('ref_axis',(0.,0.,1.));
#17179=DIRECTION('',(-1.,0.,0.));
#17180=DIRECTION('',(-1.,0.,0.));
#17181=DIRECTION('center_axis',(0.,0.,-1.));
#17182=DIRECTION('ref_axis',(-1.,0.,0.));
#17183=DIRECTION('',(0.,1.,0.));
#17184=DIRECTION('',(-1.,0.,0.));
#17185=DIRECTION('',(0.,-1.,0.));
#17186=DIRECTION('',(1.,0.,0.));
#17187=DIRECTION('center_axis',(0.,0.,-1.));
#17188=DIRECTION('ref_axis',(-1.,0.,0.));
#17189=DIRECTION('',(-1.,0.,0.));
#17190=DIRECTION('',(0.,1.,0.));
#17191=DIRECTION('',(1.,0.,0.));
#17192=DIRECTION('',(0.,-1.,0.));
#17193=DIRECTION('center_axis',(1.,0.,0.));
#17194=DIRECTION('ref_axis',(0.,0.,-1.));
#17195=DIRECTION('',(0.,0.,1.));
#17196=DIRECTION('',(0.,0.,1.));
#17197=DIRECTION('center_axis',(0.,-1.,0.));
#17198=DIRECTION('ref_axis',(0.,0.,-1.));
#17199=DIRECTION('',(0.,0.,1.));
#17200=DIRECTION('center_axis',(-1.,0.,0.));
#17201=DIRECTION('ref_axis',(0.,0.,1.));
#17202=DIRECTION('',(0.,0.,1.));
#17203=DIRECTION('center_axis',(0.,1.,0.));
#17204=DIRECTION('ref_axis',(0.,0.,1.));
#17205=DIRECTION('center_axis',(0.,0.,-1.));
#17206=DIRECTION('ref_axis',(-1.,0.,0.));
#17207=DIRECTION('',(0.,-1.,0.));
#17208=DIRECTION('',(-1.,0.,0.));
#17209=DIRECTION('',(0.,-1.,0.));
#17210=DIRECTION('',(-1.,0.,0.));
#17211=DIRECTION('center_axis',(0.,1.,9.62873847203288E-17));
#17212=DIRECTION('ref_axis',(0.,-9.62873847203288E-17,1.));
#17213=DIRECTION('',(0.,9.62873847203288E-17,-1.));
#17214=DIRECTION('',(-1.,0.,0.));
#17215=DIRECTION('',(0.,9.62873847203288E-17,-1.));
#17216=DIRECTION('center_axis',(-1.,0.,0.));
#17217=DIRECTION('ref_axis',(0.,0.,1.));
#17218=DIRECTION('center_axis',(-1.,0.,0.));
#17219=DIRECTION('ref_axis',(0.,0.,-1.));
#17220=DIRECTION('',(-1.,0.,0.));
#17221=DIRECTION('center_axis',(-1.,0.,0.));
#17222=DIRECTION('ref_axis',(0.,0.,-1.));
#17223=DIRECTION('center_axis',(0.,1.,7.93016446160826E-17));
#17224=DIRECTION('ref_axis',(0.,-7.93016446160826E-17,1.));
#17225=DIRECTION('',(0.,7.93016446160826E-17,-1.));
#17226=DIRECTION('',(-1.,0.,0.));
#17227=DIRECTION('',(0.,7.93016446160826E-17,-1.));
#17228=DIRECTION('center_axis',(0.,0.,1.));
#17229=DIRECTION('ref_axis',(1.,0.,0.));
#17230=DIRECTION('',(0.,1.,0.));
#17231=DIRECTION('',(-1.,0.,0.));
#17232=DIRECTION('',(0.,1.,0.));
#17233=DIRECTION('center_axis',(0.,-1.,0.));
#17234=DIRECTION('ref_axis',(0.,0.,-1.));
#17235=DIRECTION('',(0.,0.,1.));
#17236=DIRECTION('',(0.,0.,1.));
#17237=DIRECTION('center_axis',(1.,0.,0.));
#17238=DIRECTION('ref_axis',(0.,0.,-1.));
#17239=DIRECTION('center_axis',(1.,0.,0.));
#17240=DIRECTION('ref_axis',(0.,0.,-1.));
#17241=DIRECTION('center_axis',(0.,0.,-1.));
#17242=DIRECTION('ref_axis',(1.,0.,0.));
#17243=DIRECTION('',(0.,-1.,0.));
#17244=DIRECTION('',(1.,0.,0.));
#17245=DIRECTION('',(0.,-1.,0.));
#17246=DIRECTION('',(1.,0.,0.));
#17247=DIRECTION('center_axis',(0.,1.,9.62873847203288E-17));
#17248=DIRECTION('ref_axis',(0.,-9.62873847203288E-17,1.));
#17249=DIRECTION('',(0.,9.62873847203288E-17,-1.));
#17250=DIRECTION('',(0.,9.62873847203288E-17,-1.));
#17251=DIRECTION('',(1.,0.,0.));
#17252=DIRECTION('center_axis',(1.,0.,0.));
#17253=DIRECTION('ref_axis',(0.,0.,1.));
#17254=DIRECTION('center_axis',(-1.,0.,0.));
#17255=DIRECTION('ref_axis',(0.,0.,-1.));
#17256=DIRECTION('center_axis',(-1.,0.,0.));
#17257=DIRECTION('ref_axis',(0.,0.,-1.));
#17258=DIRECTION('',(1.,0.,0.));
#17259=DIRECTION('center_axis',(0.,1.,7.93016446160826E-17));
#17260=DIRECTION('ref_axis',(0.,-7.93016446160826E-17,1.));
#17261=DIRECTION('',(0.,7.93016446160826E-17,-1.));
#17262=DIRECTION('',(0.,7.93016446160826E-17,-1.));
#17263=DIRECTION('',(1.,0.,0.));
#17264=DIRECTION('center_axis',(0.,0.,1.));
#17265=DIRECTION('ref_axis',(-1.,0.,0.));
#17266=DIRECTION('',(0.,1.,0.));
#17267=DIRECTION('',(0.,1.,0.));
#17268=DIRECTION('',(1.,0.,0.));
#17269=DIRECTION('center_axis',(0.,-1.,0.));
#17270=DIRECTION('ref_axis',(0.,0.,-1.));
#17271=DIRECTION('',(0.,0.,1.));
#17272=DIRECTION('',(0.,0.,1.));
#17273=DIRECTION('center_axis',(-1.,0.,0.));
#17274=DIRECTION('ref_axis',(0.,0.,-1.));
#17275=DIRECTION('center_axis',(-1.,0.,0.));
#17276=DIRECTION('ref_axis',(0.,0.,-1.));
#17277=DIRECTION('center_axis',(0.,-1.,0.));
#17278=DIRECTION('ref_axis',(0.,0.,-1.));
#17279=DIRECTION('center_axis',(0.,1.,0.));
#17280=DIRECTION('ref_axis',(0.,0.,1.));
#17281=DIRECTION('',(0.,-1.,0.));
#17282=DIRECTION('center_axis',(0.,1.,0.));
#17283=DIRECTION('ref_axis',(0.,0.,1.));
#17284=DIRECTION('center_axis',(0.,-1.,0.));
#17285=DIRECTION('ref_axis',(0.,0.,-1.));
#17286=DIRECTION('center_axis',(0.,1.,0.));
#17287=DIRECTION('ref_axis',(0.,0.,1.));
#17288=DIRECTION('',(0.,-1.,0.));
#17289=DIRECTION('center_axis',(0.,1.,0.));
#17290=DIRECTION('ref_axis',(0.,0.,1.));
#17291=DIRECTION('center_axis',(0.,-1.,0.));
#17292=DIRECTION('ref_axis',(0.,0.,-1.));
#17293=DIRECTION('center_axis',(0.,1.,0.));
#17294=DIRECTION('ref_axis',(0.,0.,1.));
#17295=DIRECTION('',(0.,-1.,0.));
#17296=DIRECTION('center_axis',(0.,1.,0.));
#17297=DIRECTION('ref_axis',(0.,0.,1.));
#17298=DIRECTION('center_axis',(0.,-1.,0.));
#17299=DIRECTION('ref_axis',(0.,0.,-1.));
#17300=DIRECTION('center_axis',(0.,1.,0.));
#17301=DIRECTION('ref_axis',(0.,0.,1.));
#17302=DIRECTION('',(0.,-1.,0.));
#17303=DIRECTION('center_axis',(0.,1.,0.));
#17304=DIRECTION('ref_axis',(0.,0.,1.));
#17305=DIRECTION('center_axis',(0.,-1.,0.));
#17306=DIRECTION('ref_axis',(0.,0.,-1.));
#17307=DIRECTION('center_axis',(0.,1.,0.));
#17308=DIRECTION('ref_axis',(0.,0.,1.));
#17309=DIRECTION('',(0.,-1.,0.));
#17310=DIRECTION('center_axis',(0.,1.,0.));
#17311=DIRECTION('ref_axis',(0.,0.,1.));
#17312=DIRECTION('center_axis',(0.,-1.,0.));
#17313=DIRECTION('ref_axis',(0.,0.,-1.));
#17314=DIRECTION('center_axis',(0.,1.,0.));
#17315=DIRECTION('ref_axis',(0.,0.,1.));
#17316=DIRECTION('',(0.,-1.,0.));
#17317=DIRECTION('center_axis',(0.,1.,0.));
#17318=DIRECTION('ref_axis',(0.,0.,1.));
#17319=DIRECTION('center_axis',(0.,1.,0.));
#17320=DIRECTION('ref_axis',(0.,0.,1.));
#17321=DIRECTION('',(0.,0.,1.));
#17322=DIRECTION('',(1.,0.,-1.87133061054672E-16));
#17323=DIRECTION('',(0.,0.,-1.));
#17324=DIRECTION('',(-1.,0.,1.83697019872103E-16));
#17325=DIRECTION('center_axis',(0.,1.,0.));
#17326=DIRECTION('ref_axis',(0.,0.,1.));
#17327=DIRECTION('',(0.,0.,1.));
#17328=DIRECTION('',(-1.,0.,1.83697019872103E-16));
#17329=DIRECTION('',(0.,0.,-1.));
#17330=DIRECTION('',(1.,0.,-1.87133061054672E-16));
#17331=DIRECTION('center_axis',(1.,0.,0.));
#17332=DIRECTION('ref_axis',(0.,0.,-1.));
#17333=DIRECTION('',(0.,-1.,0.));
#17334=DIRECTION('',(0.,-1.,0.));
#17335=DIRECTION('center_axis',(-1.87133061054672E-16,0.,-1.));
#17336=DIRECTION('ref_axis',(-1.,0.,1.87133061054672E-16));
#17337=DIRECTION('',(0.,-1.,0.));
#17338=DIRECTION('center_axis',(-1.,0.,0.));
#17339=DIRECTION('ref_axis',(0.,0.,1.));
#17340=DIRECTION('',(0.,-1.,0.));
#17341=DIRECTION('center_axis',(1.83697019872103E-16,0.,1.));
#17342=DIRECTION('ref_axis',(1.,0.,-1.83697019872103E-16));
#17343=DIRECTION('center_axis',(0.,1.,0.));
#17344=DIRECTION('ref_axis',(0.,0.,1.));
#17345=DIRECTION('center_axis',(0.,1.,0.));
#17346=DIRECTION('ref_axis',(0.,0.,1.));
#17347=DIRECTION('',(0.,1.,0.));
#17348=DIRECTION('center_axis',(0.,1.,0.));
#17349=DIRECTION('ref_axis',(0.,0.,1.));
#17350=DIRECTION('center_axis',(0.,1.,0.));
#17351=DIRECTION('ref_axis',(0.,0.,1.));
#17352=DIRECTION('center_axis',(0.,1.,0.));
#17353=DIRECTION('ref_axis',(0.,0.,1.));
#17354=DIRECTION('',(0.,1.,0.));
#17355=DIRECTION('center_axis',(0.,1.,0.));
#17356=DIRECTION('ref_axis',(0.,0.,1.));
#17357=DIRECTION('center_axis',(0.,1.,0.));
#17358=DIRECTION('ref_axis',(0.,0.,1.));
#17359=DIRECTION('center_axis',(0.,1.,0.));
#17360=DIRECTION('ref_axis',(0.,0.,1.));
#17361=DIRECTION('',(0.,1.,0.));
#17362=DIRECTION('center_axis',(0.,1.,0.));
#17363=DIRECTION('ref_axis',(0.,0.,1.));
#17364=DIRECTION('center_axis',(0.,1.,0.));
#17365=DIRECTION('ref_axis',(0.,0.,1.));
#17366=DIRECTION('center_axis',(0.,1.,0.));
#17367=DIRECTION('ref_axis',(0.,0.,1.));
#17368=DIRECTION('',(0.,1.,0.));
#17369=DIRECTION('center_axis',(0.,1.,0.));
#17370=DIRECTION('ref_axis',(0.,0.,1.));
#17371=DIRECTION('center_axis',(0.,1.,0.));
#17372=DIRECTION('ref_axis',(0.,0.,1.));
#17373=DIRECTION('center_axis',(0.,1.,0.));
#17374=DIRECTION('ref_axis',(0.,0.,1.));
#17375=DIRECTION('',(0.,1.,0.));
#17376=DIRECTION('center_axis',(0.,1.,0.));
#17377=DIRECTION('ref_axis',(0.,0.,1.));
#17378=DIRECTION('center_axis',(-1.,0.,0.));
#17379=DIRECTION('ref_axis',(0.,0.,1.));
#17380=DIRECTION('',(0.,0.,1.));
#17381=DIRECTION('',(0.,1.,0.));
#17382=DIRECTION('',(0.,0.,1.));
#17383=DIRECTION('',(0.,1.,0.));
#17384=DIRECTION('center_axis',(0.,0.,-1.));
#17385=DIRECTION('ref_axis',(-1.,0.,0.));
#17386=DIRECTION('',(-1.,0.,0.));
#17387=DIRECTION('',(0.,1.,0.));
#17388=DIRECTION('',(-1.,0.,0.));
#17389=DIRECTION('center_axis',(1.,0.,0.));
#17390=DIRECTION('ref_axis',(0.,0.,-1.));
#17391=DIRECTION('',(0.,0.,-1.));
#17392=DIRECTION('',(0.,1.,0.));
#17393=DIRECTION('',(0.,0.,-1.));
#17394=DIRECTION('center_axis',(0.,0.,1.));
#17395=DIRECTION('ref_axis',(1.,0.,0.));
#17396=DIRECTION('',(1.,0.,0.));
#17397=DIRECTION('',(1.,0.,0.));
#17398=DIRECTION('center_axis',(0.,-1.,0.));
#17399=DIRECTION('ref_axis',(0.,0.,-1.));
#17400=DIRECTION('center_axis',(0.,-1.,0.));
#17401=DIRECTION('ref_axis',(0.,0.,-1.));
#17402=DIRECTION('center_axis',(0.,1.,0.));
#17403=DIRECTION('ref_axis',(0.,0.,1.));
#17404=DIRECTION('center_axis',(0.,-1.,0.));
#17405=DIRECTION('ref_axis',(0.,0.,1.));
#17406=DIRECTION('',(0.,1.,0.));
#17407=DIRECTION('center_axis',(0.,-1.,0.));
#17408=DIRECTION('ref_axis',(0.,0.,1.));
#17409=DIRECTION('center_axis',(0.,1.,0.));
#17410=DIRECTION('ref_axis',(0.,0.,1.));
#17411=DIRECTION('center_axis',(0.,-1.,0.));
#17412=DIRECTION('ref_axis',(0.,0.,1.));
#17413=DIRECTION('',(0.,1.,0.));
#17414=DIRECTION('center_axis',(0.,-1.,0.));
#17415=DIRECTION('ref_axis',(0.,0.,1.));
#17416=DIRECTION('center_axis',(0.,1.,0.));
#17417=DIRECTION('ref_axis',(0.,0.,1.));
#17418=DIRECTION('center_axis',(0.,-1.,0.));
#17419=DIRECTION('ref_axis',(0.,0.,1.));
#17420=DIRECTION('',(0.,1.,0.));
#17421=DIRECTION('center_axis',(0.,-1.,0.));
#17422=DIRECTION('ref_axis',(0.,0.,1.));
#17423=DIRECTION('center_axis',(0.,1.,0.));
#17424=DIRECTION('ref_axis',(0.,0.,1.));
#17425=DIRECTION('center_axis',(0.,-1.,0.));
#17426=DIRECTION('ref_axis',(0.,0.,1.));
#17427=DIRECTION('',(0.,1.,0.));
#17428=DIRECTION('center_axis',(0.,-1.,0.));
#17429=DIRECTION('ref_axis',(0.,0.,1.));
#17430=DIRECTION('center_axis',(0.,1.,0.));
#17431=DIRECTION('ref_axis',(0.,0.,1.));
#17432=DIRECTION('center_axis',(0.,-1.,0.));
#17433=DIRECTION('ref_axis',(0.,0.,1.));
#17434=DIRECTION('',(0.,1.,0.));
#17435=DIRECTION('center_axis',(0.,-1.,0.));
#17436=DIRECTION('ref_axis',(0.,0.,1.));
#17437=DIRECTION('center_axis',(1.,0.,0.));
#17438=DIRECTION('ref_axis',(0.,0.,1.));
#17439=DIRECTION('',(0.,0.,1.));
#17440=DIRECTION('',(0.,1.,0.));
#17441=DIRECTION('',(0.,0.,1.));
#17442=DIRECTION('',(0.,1.,0.));
#17443=DIRECTION('center_axis',(0.,0.,-1.));
#17444=DIRECTION('ref_axis',(1.,0.,0.));
#17445=DIRECTION('',(1.,0.,0.));
#17446=DIRECTION('',(1.,0.,0.));
#17447=DIRECTION('',(0.,1.,0.));
#17448=DIRECTION('center_axis',(-1.,0.,0.));
#17449=DIRECTION('ref_axis',(0.,0.,-1.));
#17450=DIRECTION('',(0.,0.,-1.));
#17451=DIRECTION('',(0.,0.,-1.));
#17452=DIRECTION('',(0.,1.,0.));
#17453=DIRECTION('center_axis',(0.,0.,1.));
#17454=DIRECTION('ref_axis',(-1.,0.,0.));
#17455=DIRECTION('',(-1.,0.,0.));
#17456=DIRECTION('',(-1.,0.,0.));
#17457=DIRECTION('center_axis',(0.,-1.,0.));
#17458=DIRECTION('ref_axis',(0.,0.,-1.));
#17459=DIRECTION('center_axis',(0.,-1.,0.));
#17460=DIRECTION('ref_axis',(0.,0.,-1.));
#17461=DIRECTION('center_axis',(-1.87133061054672E-16,0.,-1.));
#17462=DIRECTION('ref_axis',(-1.,0.,1.87133061054672E-16));
#17463=DIRECTION('',(-1.,0.,1.87133061054672E-16));
#17464=DIRECTION('',(0.,1.,0.));
#17465=DIRECTION('',(-1.,0.,1.87133061054672E-16));
#17466=DIRECTION('',(0.,1.,0.));
#17467=DIRECTION('center_axis',(1.,0.,0.));
#17468=DIRECTION('ref_axis',(0.,0.,-1.));
#17469=DIRECTION('',(0.,0.,-1.));
#17470=DIRECTION('',(0.,1.,0.));
#17471=DIRECTION('',(0.,0.,-1.));
#17472=DIRECTION('center_axis',(1.83697019872103E-16,0.,1.));
#17473=DIRECTION('ref_axis',(1.,0.,-1.83697019872103E-16));
#17474=DIRECTION('',(1.,0.,-1.83697019872103E-16));
#17475=DIRECTION('',(0.,1.,0.));
#17476=DIRECTION('',(1.,0.,-1.83697019872103E-16));
#17477=DIRECTION('center_axis',(-1.,0.,0.));
#17478=DIRECTION('ref_axis',(0.,0.,1.));
#17479=DIRECTION('',(0.,0.,1.));
#17480=DIRECTION('',(0.,0.,1.));
#17481=DIRECTION('center_axis',(0.,-1.,0.));
#17482=DIRECTION('ref_axis',(0.,0.,-1.));
#17483=DIRECTION('center_axis',(0.,-1.,0.));
#17484=DIRECTION('ref_axis',(0.,0.,-1.));
#17485=DIRECTION('center_axis',(-1.,0.,0.));
#17486=DIRECTION('ref_axis',(0.,0.,1.));
#17487=DIRECTION('',(0.,-1.18360663606093E-16,1.));
#17488=DIRECTION('',(0.,1.,9.62873847203288E-17));
#17489=DIRECTION('',(0.,-1.18360663606093E-16,1.));
#17490=DIRECTION('',(0.,1.,9.62873847203288E-17));
#17491=DIRECTION('center_axis',(-3.7224019040034E-16,9.62873847203288E-17,
-1.));
#17492=DIRECTION('ref_axis',(-1.,-2.72359540441036E-48,3.7224019040034E-16));
#17493=DIRECTION('',(-1.,0.,3.7224019040034E-16));
#17494=DIRECTION('',(0.,1.,9.62873847203288E-17));
#17495=DIRECTION('',(-1.,0.,3.7224019040034E-16));
#17496=DIRECTION('center_axis',(1.,0.,0.));
#17497=DIRECTION('ref_axis',(0.,0.,-1.));
#17498=DIRECTION('',(0.,1.18360663606093E-16,-1.));
#17499=DIRECTION('',(0.,1.,9.62873847203288E-17));
#17500=DIRECTION('',(0.,1.18360663606093E-16,-1.));
#17501=DIRECTION('center_axis',(0.,-9.62873847203288E-17,1.));
#17502=DIRECTION('ref_axis',(0.,-1.,-9.62873847203289E-17));
#17503=DIRECTION('',(1.,0.,0.));
#17504=DIRECTION('',(1.,0.,0.));
#17505=DIRECTION('center_axis',(0.,1.,1.18360663606093E-16));
#17506=DIRECTION('ref_axis',(0.,-1.18360663606093E-16,1.));
#17507=DIRECTION('center_axis',(0.,1.,1.18360663606093E-16));
#17508=DIRECTION('ref_axis',(0.,-1.18360663606093E-16,1.));
#17509=DIRECTION('center_axis',(1.,0.,0.));
#17510=DIRECTION('ref_axis',(0.,0.,1.));
#17511=DIRECTION('',(0.,-1.18360663606093E-16,1.));
#17512=DIRECTION('',(0.,1.,9.62873847203288E-17));
#17513=DIRECTION('',(0.,-1.18360663606093E-16,1.));
#17514=DIRECTION('',(0.,1.,9.62873847203288E-17));
#17515=DIRECTION('center_axis',(3.7224019040034E-16,9.62873847203288E-17,
-1.));
#17516=DIRECTION('ref_axis',(1.,-2.72359540441036E-48,3.7224019040034E-16));
#17517=DIRECTION('',(1.,0.,3.7224019040034E-16));
#17518=DIRECTION('',(1.,0.,3.7224019040034E-16));
#17519=DIRECTION('',(0.,1.,9.62873847203288E-17));
#17520=DIRECTION('center_axis',(-1.,0.,0.));
#17521=DIRECTION('ref_axis',(0.,0.,-1.));
#17522=DIRECTION('',(0.,1.18360663606093E-16,-1.));
#17523=DIRECTION('',(0.,1.18360663606093E-16,-1.));
#17524=DIRECTION('',(0.,1.,9.62873847203288E-17));
#17525=DIRECTION('center_axis',(0.,-9.62873847203288E-17,1.));
#17526=DIRECTION('ref_axis',(0.,-1.,-9.62873847203289E-17));
#17527=DIRECTION('',(-1.,0.,0.));
#17528=DIRECTION('',(-1.,0.,0.));
#17529=DIRECTION('center_axis',(0.,1.,1.18360663606093E-16));
#17530=DIRECTION('ref_axis',(0.,-1.18360663606093E-16,1.));
#17531=DIRECTION('center_axis',(0.,1.,1.18360663606093E-16));
#17532=DIRECTION('ref_axis',(0.,-1.18360663606093E-16,1.));
#21310=CARTESIAN_POINT('',(0.,0.,0.));
#21311=CARTESIAN_POINT('Origin',(400.,-261.,-12.7));
#21312=CARTESIAN_POINT('',(400.,-261.,0.));
#21313=CARTESIAN_POINT('',(400.,261.,0.));
#21314=CARTESIAN_POINT('',(400.,-261.,0.));
#21315=CARTESIAN_POINT('',(400.,-261.,-12.7));
#21316=CARTESIAN_POINT('',(400.,-261.,-12.7));
#21317=CARTESIAN_POINT('',(400.,261.,-12.7));
#21318=CARTESIAN_POINT('',(400.,-261.,-12.7));
#21319=CARTESIAN_POINT('',(400.,261.,-12.7));
#21320=CARTESIAN_POINT('Origin',(-400.,-261.,-12.7));
#21321=CARTESIAN_POINT('',(-400.,-261.,0.));
#21322=CARTESIAN_POINT('',(-400.,-261.,0.));
#21323=CARTESIAN_POINT('',(-400.,-261.,-12.7));
#21324=CARTESIAN_POINT('',(-400.,-261.,-12.7));
#21325=CARTESIAN_POINT('',(-400.,-261.,-12.7));
#21326=CARTESIAN_POINT('Origin',(-400.,-261.,-12.7));
#21327=CARTESIAN_POINT('',(-400.,261.,0.));
#21328=CARTESIAN_POINT('',(-400.,-261.,0.));
#21329=CARTESIAN_POINT('',(-400.,261.,-12.7));
#21330=CARTESIAN_POINT('',(-400.,261.,-12.7));
#21331=CARTESIAN_POINT('',(-400.,-261.,-12.7));
#21332=CARTESIAN_POINT('Origin',(-400.,261.,-12.7));
#21333=CARTESIAN_POINT('',(-400.,261.,0.));
#21334=CARTESIAN_POINT('',(-400.,261.,-12.7));
#21335=CARTESIAN_POINT('Origin',(0.,0.,-12.7));
#21336=CARTESIAN_POINT('',(250.,-200.,-12.7));
#21337=CARTESIAN_POINT('',(250.,200.,-12.7));
#21338=CARTESIAN_POINT('',(250.,-200.,-12.7));
#21339=CARTESIAN_POINT('',(-250.,200.,-12.7));
#21340=CARTESIAN_POINT('',(-250.,200.,-12.7));
#21341=CARTESIAN_POINT('',(-250.,-200.,-12.7));
#21342=CARTESIAN_POINT('',(-250.,-200.,-12.7));
#21343=CARTESIAN_POINT('',(-250.,-200.,-12.7));
#21344=CARTESIAN_POINT('Origin',(0.,0.,0.));
#21345=CARTESIAN_POINT('',(250.,200.,0.));
#21346=CARTESIAN_POINT('',(-250.,200.,0.));
#21347=CARTESIAN_POINT('',(-250.,200.,0.));
#21348=CARTESIAN_POINT('',(250.,-200.,0.));
#21349=CARTESIAN_POINT('',(250.,-200.,0.));
#21350=CARTESIAN_POINT('',(-250.,-200.,0.));
#21351=CARTESIAN_POINT('',(-250.,-200.,0.));
#21352=CARTESIAN_POINT('',(-250.,-200.,0.));
#21353=CARTESIAN_POINT('Origin',(250.,-200.,-12.7));
#21354=CARTESIAN_POINT('',(250.,200.,-12.7));
#21355=CARTESIAN_POINT('',(250.,-200.,-12.7));
#21356=CARTESIAN_POINT('Origin',(-250.,-200.,-12.7));
#21357=CARTESIAN_POINT('',(-250.,-200.,-12.7));
#21358=CARTESIAN_POINT('Origin',(-250.,-200.,-12.7));
#21359=CARTESIAN_POINT('',(-250.,200.,-12.7));
#21360=CARTESIAN_POINT('Origin',(-250.,200.,-12.7));
#21361=CARTESIAN_POINT('Origin',(412.7,261.,-12.7));
#21362=CARTESIAN_POINT('',(400.,261.,-12.7));
#21363=CARTESIAN_POINT('',(400.,-261.,-12.7));
#21364=CARTESIAN_POINT('',(400.,261.,-12.7));
#21365=CARTESIAN_POINT('',(412.7,-261.,-12.7));
#21366=CARTESIAN_POINT('',(412.7,-261.,-12.7));
#21367=CARTESIAN_POINT('',(412.7,261.,-12.7));
#21368=CARTESIAN_POINT('',(412.7,261.,-12.7));
#21369=CARTESIAN_POINT('',(412.7,261.,-12.7));
#21370=CARTESIAN_POINT('Origin',(412.7,-261.,-589.215307716505));
#21371=CARTESIAN_POINT('',(400.,-261.,-589.215307716505));
#21372=CARTESIAN_POINT('',(400.,-261.,-589.215307716505));
#21373=CARTESIAN_POINT('',(412.7,-261.,-589.215307716505));
#21374=CARTESIAN_POINT('',(412.7,-261.,-589.215307716505));
#21375=CARTESIAN_POINT('',(412.7,-261.,-589.215307716505));
#21376=CARTESIAN_POINT('Origin',(412.7,-276.,-662.7));
#21377=CARTESIAN_POINT('',(400.,-201.,-662.7));
#21378=CARTESIAN_POINT('Origin',(400.,-276.,-662.7));
#21379=CARTESIAN_POINT('',(412.7,-201.,-662.7));
#21380=CARTESIAN_POINT('',(412.7,-201.,-662.7));
#21381=CARTESIAN_POINT('Origin',(412.7,-276.,-662.7));
#21382=CARTESIAN_POINT('Origin',(412.7,-201.,-1012.7));
#21383=CARTESIAN_POINT('',(400.,-201.,-1012.7));
#21384=CARTESIAN_POINT('',(400.,-201.,-1012.7));
#21385=CARTESIAN_POINT('',(412.7,-201.,-1012.7));
#21386=CARTESIAN_POINT('',(412.7,-201.,-1012.7));
#21387=CARTESIAN_POINT('',(412.7,-201.,-1012.7));
#21388=CARTESIAN_POINT('Origin',(412.7,261.,-1012.7));
#21389=CARTESIAN_POINT('',(400.,261.,-1012.7));
#21390=CARTESIAN_POINT('',(400.,261.,-1012.7));
#21391=CARTESIAN_POINT('',(412.7,261.,-1012.7));
#21392=CARTESIAN_POINT('',(412.7,261.,-1012.7));
#21393=CARTESIAN_POINT('',(412.7,261.,-1012.7));
#21394=CARTESIAN_POINT('Origin',(412.7,261.,-12.7));
#21395=CARTESIAN_POINT('',(400.,261.,-12.7));
#21396=CARTESIAN_POINT('',(412.7,261.,-12.7));
#21397=CARTESIAN_POINT('Origin',(412.7,-276.,-662.7));
#21398=CARTESIAN_POINT('Origin',(400.,-276.,-662.7));
#21399=CARTESIAN_POINT('Origin',(-412.7,261.,-12.7));
#21400=CARTESIAN_POINT('',(-400.,261.,-12.7));
#21401=CARTESIAN_POINT('',(-400.,-261.,-12.7));
#21402=CARTESIAN_POINT('',(-400.,261.,-12.7));
#21403=CARTESIAN_POINT('',(-412.7,261.,-12.7));
#21404=CARTESIAN_POINT('',(-412.7,261.,-12.7));
#21405=CARTESIAN_POINT('',(-412.7,-261.,-12.7));
#21406=CARTESIAN_POINT('',(-412.7,261.,-12.7));
#21407=CARTESIAN_POINT('',(-412.7,-261.,-12.7));
#21408=CARTESIAN_POINT('Origin',(-412.7,-261.,-589.215307716505));
#21409=CARTESIAN_POINT('',(-400.,-261.,-589.215307716505));
#21410=CARTESIAN_POINT('',(-400.,-261.,-589.215307716505));
#21411=CARTESIAN_POINT('',(-412.7,-261.,-589.215307716505));
#21412=CARTESIAN_POINT('',(-412.7,-261.,-589.215307716505));
#21413=CARTESIAN_POINT('',(-412.7,-261.,-589.215307716505));
#21414=CARTESIAN_POINT('Origin',(-412.7,-276.,-662.7));
#21415=CARTESIAN_POINT('',(-400.,-201.,-662.7));
#21416=CARTESIAN_POINT('Origin',(-400.,-276.,-662.7));
#21417=CARTESIAN_POINT('',(-412.7,-201.,-662.7));
#21418=CARTESIAN_POINT('Origin',(-412.7,-276.,-662.7));
#21419=CARTESIAN_POINT('',(-412.7,-201.,-662.7));
#21420=CARTESIAN_POINT('Origin',(-412.7,-201.,-1012.7));
#21421=CARTESIAN_POINT('',(-400.,-201.,-1012.7));
#21422=CARTESIAN_POINT('',(-400.,-201.,-1012.7));
#21423=CARTESIAN_POINT('',(-412.7,-201.,-1012.7));
#21424=CARTESIAN_POINT('',(-412.7,-201.,-1012.7));
#21425=CARTESIAN_POINT('',(-412.7,-201.,-1012.7));
#21426=CARTESIAN_POINT('Origin',(-412.7,261.,-1012.7));
#21427=CARTESIAN_POINT('',(-400.,261.,-1012.7));
#21428=CARTESIAN_POINT('',(-400.,261.,-1012.7));
#21429=CARTESIAN_POINT('',(-412.7,261.,-1012.7));
#21430=CARTESIAN_POINT('',(-412.7,261.,-1012.7));
#21431=CARTESIAN_POINT('',(-412.7,261.,-1012.7));
#21432=CARTESIAN_POINT('Origin',(-412.7,261.,-12.7));
#21433=CARTESIAN_POINT('',(-400.,261.,-12.7));
#21434=CARTESIAN_POINT('',(-412.7,261.,-12.7));
#21435=CARTESIAN_POINT('Origin',(-412.7,-276.,-662.7));
#21436=CARTESIAN_POINT('Origin',(-400.,-276.,-662.7));
#21437=CARTESIAN_POINT('Origin',(442.5,276.875,30.));
#21438=CARTESIAN_POINT('',(442.5,276.875,39.));
#21439=CARTESIAN_POINT('Origin',(442.5,276.875,30.));
#21440=CARTESIAN_POINT('',(442.5,261.,39.));
#21441=CARTESIAN_POINT('',(442.5,276.875,39.));
#21442=CARTESIAN_POINT('Origin',(442.5,261.,30.));
#21443=CARTESIAN_POINT('Origin',(265.5,276.875,30.));
#21444=CARTESIAN_POINT('',(265.5,276.875,39.));
#21445=CARTESIAN_POINT('Origin',(265.5,276.875,30.));
#21446=CARTESIAN_POINT('',(265.5,261.,39.));
#21447=CARTESIAN_POINT('',(265.5,276.875,39.));
#21448=CARTESIAN_POINT('Origin',(265.5,261.,30.));
#21449=CARTESIAN_POINT('Origin',(88.4999999999999,276.875,30.));
#21450=CARTESIAN_POINT('',(88.4999999999999,276.875,39.));
#21451=CARTESIAN_POINT('Origin',(88.4999999999999,276.875,30.));
#21452=CARTESIAN_POINT('',(88.4999999999999,261.,39.));
#21453=CARTESIAN_POINT('',(88.4999999999999,276.875,39.));
#21454=CARTESIAN_POINT('Origin',(88.4999999999999,261.,30.));
#21455=CARTESIAN_POINT('Origin',(-88.5,276.875,30.));
#21456=CARTESIAN_POINT('',(-88.5,276.875,39.));
#21457=CARTESIAN_POINT('Origin',(-88.5,276.875,30.));
#21458=CARTESIAN_POINT('',(-88.5,261.,39.));
#21459=CARTESIAN_POINT('',(-88.5,276.875,39.));
#21460=CARTESIAN_POINT('Origin',(-88.5,261.,30.));
#21461=CARTESIAN_POINT('Origin',(-265.5,276.875,30.));
#21462=CARTESIAN_POINT('',(-265.5,276.875,39.));
#21463=CARTESIAN_POINT('Origin',(-265.5,276.875,30.));
#21464=CARTESIAN_POINT('',(-265.5,261.,39.));
#21465=CARTESIAN_POINT('',(-265.5,276.875,39.));
#21466=CARTESIAN_POINT('Origin',(-265.5,261.,30.));
#21467=CARTESIAN_POINT('Origin',(-442.5,276.875,30.));
#21468=CARTESIAN_POINT('',(-442.5,276.875,39.));
#21469=CARTESIAN_POINT('Origin',(-442.5,276.875,30.));
#21470=CARTESIAN_POINT('',(-442.5,261.,39.));
#21471=CARTESIAN_POINT('',(-442.5,276.875,39.));
#21472=CARTESIAN_POINT('Origin',(-442.5,261.,30.));
#21473=CARTESIAN_POINT('Origin',(0.,276.875,0.));
#21474=CARTESIAN_POINT('',(-463.5,276.875,0.));
#21475=CARTESIAN_POINT('',(-463.5,276.875,51.));
#21476=CARTESIAN_POINT('',(-463.5,276.875,0.));
#21477=CARTESIAN_POINT('',(463.5,276.875,50.9999999999998));
#21478=CARTESIAN_POINT('',(-463.5,276.875,51.));
#21479=CARTESIAN_POINT('',(463.5,276.875,-1.70287137421439E-13));
#21480=CARTESIAN_POINT('',(463.5,276.875,-1.70287137421439E-13));
#21481=CARTESIAN_POINT('',(-463.5,276.875,0.));
#21482=CARTESIAN_POINT('Origin',(0.,261.,0.));
#21483=CARTESIAN_POINT('',(-463.5,261.,0.));
#21484=CARTESIAN_POINT('',(-463.5,261.,51.));
#21485=CARTESIAN_POINT('',(-463.5,261.,0.));
#21486=CARTESIAN_POINT('',(463.5,261.,-1.70287137421439E-13));
#21487=CARTESIAN_POINT('',(-463.5,261.,0.));
#21488=CARTESIAN_POINT('',(463.5,261.,50.9999999999998));
#21489=CARTESIAN_POINT('',(463.5,261.,-1.70287137421439E-13));
#21490=CARTESIAN_POINT('',(-463.5,261.,51.));
#21491=CARTESIAN_POINT('Origin',(-463.5,276.875,0.));
#21492=CARTESIAN_POINT('',(-463.5,276.875,51.));
#21493=CARTESIAN_POINT('',(-463.5,276.875,0.));
#21494=CARTESIAN_POINT('Origin',(-463.5,276.875,51.));
#21495=CARTESIAN_POINT('',(463.5,276.875,50.9999999999998));
#21496=CARTESIAN_POINT('Origin',(463.5,276.875,-1.70287137421439E-13));
#21497=CARTESIAN_POINT('',(463.5,276.875,-1.70287137421439E-13));
#21498=CARTESIAN_POINT('Origin',(-463.5,276.875,0.));
#21499=CARTESIAN_POINT('Origin',(-442.5,261.,-170.));
#21500=CARTESIAN_POINT('',(-442.5,261.,-179.));
#21501=CARTESIAN_POINT('Origin',(-442.5,261.,-170.));
#21502=CARTESIAN_POINT('',(-442.5,276.875,-179.));
#21503=CARTESIAN_POINT('',(-442.5,261.,-179.));
#21504=CARTESIAN_POINT('Origin',(-442.5,276.875,-170.));
#21505=CARTESIAN_POINT('Origin',(-442.499999999994,261.,-370.175));
#21506=CARTESIAN_POINT('',(-442.499999999994,261.,-379.175));
#21507=CARTESIAN_POINT('Origin',(-442.499999999994,261.,-370.175));
#21508=CARTESIAN_POINT('',(-442.499999999994,276.875,-379.175));
#21509=CARTESIAN_POINT('',(-442.499999999994,261.,-379.175));
#21510=CARTESIAN_POINT('Origin',(-442.499999999994,276.875,-370.175));
#21511=CARTESIAN_POINT('Origin',(-442.499999999996,261.,-570.35));
#21512=CARTESIAN_POINT('',(-442.499999999996,261.,-579.35));
#21513=CARTESIAN_POINT('Origin',(-442.499999999996,261.,-570.35));
#21514=CARTESIAN_POINT('',(-442.499999999996,276.875,-579.35));
#21515=CARTESIAN_POINT('',(-442.499999999996,261.,-579.35));
#21516=CARTESIAN_POINT('Origin',(-442.499999999996,276.875,-570.35));
#21517=CARTESIAN_POINT('Origin',(-442.499999999998,261.,-770.525));
#21518=CARTESIAN_POINT('',(-442.499999999998,261.,-779.525));
#21519=CARTESIAN_POINT('Origin',(-442.499999999998,261.,-770.525));
#21520=CARTESIAN_POINT('',(-442.499999999998,276.875,-779.525));
#21521=CARTESIAN_POINT('',(-442.499999999998,261.,-779.525));
#21522=CARTESIAN_POINT('Origin',(-442.499999999998,276.875,-770.525));
#21523=CARTESIAN_POINT('Origin',(-442.5,261.,-970.7));
#21524=CARTESIAN_POINT('',(-442.5,261.,-979.7));
#21525=CARTESIAN_POINT('Origin',(-442.5,261.,-970.7));
#21526=CARTESIAN_POINT('',(-442.5,276.875,-979.7));
#21527=CARTESIAN_POINT('',(-442.5,261.,-979.7));
#21528=CARTESIAN_POINT('Origin',(-442.5,276.875,-970.7));
#21529=CARTESIAN_POINT('Origin',(-463.5,261.,0.));
#21530=CARTESIAN_POINT('',(-463.5,276.875,-1012.7));
#21531=CARTESIAN_POINT('',(-463.5,276.875,0.));
#21532=CARTESIAN_POINT('',(-463.5,276.875,0.));
#21533=CARTESIAN_POINT('',(-463.5,261.,-1012.7));
#21534=CARTESIAN_POINT('',(-463.5,261.,-1012.7));
#21535=CARTESIAN_POINT('',(-463.5,261.,0.));
#21536=CARTESIAN_POINT('',(-463.5,261.,0.));
#21537=CARTESIAN_POINT('',(-463.5,261.,0.));
#21538=CARTESIAN_POINT('Origin',(-463.5,261.,-1012.7));
#21539=CARTESIAN_POINT('',(-412.7,276.875,-1012.7));
#21540=CARTESIAN_POINT('',(-463.5,276.875,-1012.7));
#21541=CARTESIAN_POINT('',(-412.7,261.,-1012.7));
#21542=CARTESIAN_POINT('',(-412.7,261.,-1012.7));
#21543=CARTESIAN_POINT('',(-463.5,261.,-1012.7));
#21544=CARTESIAN_POINT('Origin',(-412.7,261.,0.));
#21545=CARTESIAN_POINT('',(-412.7,276.875,0.));
#21546=CARTESIAN_POINT('',(-412.7,276.875,0.));
#21547=CARTESIAN_POINT('',(-412.7,261.,0.));
#21548=CARTESIAN_POINT('',(-412.7,261.,0.));
#21549=CARTESIAN_POINT('',(-412.7,261.,0.));
#21550=CARTESIAN_POINT('Origin',(-463.5,261.,0.));
#21551=CARTESIAN_POINT('',(-463.5,276.875,0.));
#21552=CARTESIAN_POINT('',(-463.5,261.,0.));
#21553=CARTESIAN_POINT('Origin',(0.,261.,0.));
#21554=CARTESIAN_POINT('Origin',(0.,276.875,0.));
#21555=CARTESIAN_POINT('Origin',(442.5,261.,-170.));
#21556=CARTESIAN_POINT('',(442.5,261.,-179.));
#21557=CARTESIAN_POINT('Origin',(442.5,261.,-170.));
#21558=CARTESIAN_POINT('',(442.5,276.875,-179.));
#21559=CARTESIAN_POINT('',(442.5,261.,-179.));
#21560=CARTESIAN_POINT('Origin',(442.5,276.875,-170.));
#21561=CARTESIAN_POINT('Origin',(442.499999999994,261.,-370.175));
#21562=CARTESIAN_POINT('',(442.499999999994,261.,-379.175));
#21563=CARTESIAN_POINT('Origin',(442.499999999994,261.,-370.175));
#21564=CARTESIAN_POINT('',(442.499999999994,276.875,-379.175));
#21565=CARTESIAN_POINT('',(442.499999999994,261.,-379.175));
#21566=CARTESIAN_POINT('Origin',(442.499999999994,276.875,-370.175));
#21567=CARTESIAN_POINT('Origin',(442.499999999996,261.,-570.35));
#21568=CARTESIAN_POINT('',(442.499999999996,261.,-579.35));
#21569=CARTESIAN_POINT('Origin',(442.499999999996,261.,-570.35));
#21570=CARTESIAN_POINT('',(442.499999999996,276.875,-579.35));
#21571=CARTESIAN_POINT('',(442.499999999996,261.,-579.35));
#21572=CARTESIAN_POINT('Origin',(442.499999999996,276.875,-570.35));
#21573=CARTESIAN_POINT('Origin',(442.499999999998,261.,-770.525));
#21574=CARTESIAN_POINT('',(442.499999999998,261.,-779.525));
#21575=CARTESIAN_POINT('Origin',(442.499999999998,261.,-770.525));
#21576=CARTESIAN_POINT('',(442.499999999998,276.875,-779.525));
#21577=CARTESIAN_POINT('',(442.499999999998,261.,-779.525));
#21578=CARTESIAN_POINT('Origin',(442.499999999998,276.875,-770.525));
#21579=CARTESIAN_POINT('Origin',(442.5,261.,-970.7));
#21580=CARTESIAN_POINT('',(442.5,261.,-979.7));
#21581=CARTESIAN_POINT('Origin',(442.5,261.,-970.7));
#21582=CARTESIAN_POINT('',(442.5,276.875,-979.7));
#21583=CARTESIAN_POINT('',(442.5,261.,-979.7));
#21584=CARTESIAN_POINT('Origin',(442.5,276.875,-970.7));
#21585=CARTESIAN_POINT('Origin',(463.5,261.,0.));
#21586=CARTESIAN_POINT('',(463.5,276.875,-1012.7));
#21587=CARTESIAN_POINT('',(463.5,276.875,0.));
#21588=CARTESIAN_POINT('',(463.5,276.875,0.));
#21589=CARTESIAN_POINT('',(463.5,261.,0.));
#21590=CARTESIAN_POINT('',(463.5,261.,0.));
#21591=CARTESIAN_POINT('',(463.5,261.,-1012.7));
#21592=CARTESIAN_POINT('',(463.5,261.,0.));
#21593=CARTESIAN_POINT('',(463.5,261.,-1012.7));
#21594=CARTESIAN_POINT('Origin',(463.5,261.,-1012.7));
#21595=CARTESIAN_POINT('',(412.7,276.875,-1012.7));
#21596=CARTESIAN_POINT('',(463.5,276.875,-1012.7));
#21597=CARTESIAN_POINT('',(412.7,261.,-1012.7));
#21598=CARTESIAN_POINT('',(463.5,261.,-1012.7));
#21599=CARTESIAN_POINT('',(412.7,261.,-1012.7));
#21600=CARTESIAN_POINT('Origin',(412.7,261.,0.));
#21601=CARTESIAN_POINT('',(412.7,276.875,0.));
#21602=CARTESIAN_POINT('',(412.7,276.875,0.));
#21603=CARTESIAN_POINT('',(412.7,261.,0.));
#21604=CARTESIAN_POINT('',(412.7,261.,0.));
#21605=CARTESIAN_POINT('',(412.7,261.,0.));
#21606=CARTESIAN_POINT('Origin',(463.5,261.,0.));
#21607=CARTESIAN_POINT('',(463.5,276.875,0.));
#21608=CARTESIAN_POINT('',(463.5,261.,0.));
#21609=CARTESIAN_POINT('Origin',(0.,261.,0.));
#21610=CARTESIAN_POINT('Origin',(0.,276.875,0.));
#21611=CARTESIAN_POINT('Origin',(463.5,-276.875,50.9999999999998));
#21612=CARTESIAN_POINT('',(463.5,-261.,50.9999999999998));
#21613=CARTESIAN_POINT('',(-463.5,-261.,51.));
#21614=CARTESIAN_POINT('',(463.5,-261.,50.9999999999998));
#21615=CARTESIAN_POINT('',(-463.5,-276.875,51.));
#21616=CARTESIAN_POINT('',(-463.5,-276.875,51.));
#21617=CARTESIAN_POINT('',(463.5,-276.875,50.9999999999998));
#21618=CARTESIAN_POINT('',(463.5,-276.875,50.9999999999998));
#21619=CARTESIAN_POINT('',(463.5,-276.875,50.9999999999998));
#21620=CARTESIAN_POINT('Origin',(-463.5,-276.875,51.));
#21621=CARTESIAN_POINT('',(-463.5,-261.,0.));
#21622=CARTESIAN_POINT('',(-463.5,-261.,51.));
#21623=CARTESIAN_POINT('',(-463.5,-276.875,0.));
#21624=CARTESIAN_POINT('',(-463.5,-276.875,0.));
#21625=CARTESIAN_POINT('',(-463.5,-276.875,51.));
#21626=CARTESIAN_POINT('Origin',(-463.5,-276.875,0.));
#21627=CARTESIAN_POINT('',(463.5,-261.,-1.70287137421439E-13));
#21628=CARTESIAN_POINT('',(-463.5,-261.,0.));
#21629=CARTESIAN_POINT('',(463.5,-276.875,-1.70287137421439E-13));
#21630=CARTESIAN_POINT('',(463.5,-276.875,-1.70287137421439E-13));
#21631=CARTESIAN_POINT('',(-463.5,-276.875,0.));
#21632=CARTESIAN_POINT('Origin',(463.5,-276.875,-1.70287137421439E-13));
#21633=CARTESIAN_POINT('',(463.5,-261.,-1.70287137421439E-13));
#21634=CARTESIAN_POINT('',(463.5,-276.875,-1.70287137421439E-13));
#21635=CARTESIAN_POINT('Origin',(0.,-276.875,0.));
#21636=CARTESIAN_POINT('Origin',(0.,-261.,0.));
#21637=CARTESIAN_POINT('Origin',(463.5,-276.875,-5.17905770564469E-14));
#21638=CARTESIAN_POINT('',(463.5,-261.,-469.));
#21639=CARTESIAN_POINT('',(463.5,-261.,-5.02620148240116E-14));
#21640=CARTESIAN_POINT('',(463.5,-261.,-5.02620148240116E-14));
#21641=CARTESIAN_POINT('',(463.5,-276.875,-5.17905770564469E-14));
#21642=CARTESIAN_POINT('',(463.5,-276.875,-5.17905770564469E-14));
#21643=CARTESIAN_POINT('',(463.5,-276.875,-469.));
#21644=CARTESIAN_POINT('',(463.5,-276.875,-5.17905770564469E-14));
#21645=CARTESIAN_POINT('',(463.5,-276.875,-469.));
#21646=CARTESIAN_POINT('Origin',(463.5,-276.875,-5.17905770564469E-14));
#21647=CARTESIAN_POINT('',(412.7,-261.,-3.13522131516744E-14));
#21648=CARTESIAN_POINT('',(463.5,-261.,-5.02620148240116E-14));
#21649=CARTESIAN_POINT('',(412.7,-276.875,-3.28807753841096E-14));
#21650=CARTESIAN_POINT('',(412.7,-276.875,-3.28807753841096E-14));
#21651=CARTESIAN_POINT('',(463.5,-276.875,-5.17905770564469E-14));
#21652=CARTESIAN_POINT('Origin',(412.7,-276.875,-3.28807753841096E-14));
#21653=CARTESIAN_POINT('',(412.7,-261.,-469.));
#21654=CARTESIAN_POINT('',(412.7,-261.,-3.13522131516744E-14));
#21655=CARTESIAN_POINT('',(412.7,-276.875,-469.));
#21656=CARTESIAN_POINT('',(412.7,-276.875,-469.));
#21657=CARTESIAN_POINT('',(412.7,-276.875,-3.28807753841096E-14));
#21658=CARTESIAN_POINT('Origin',(463.5,-276.875,-469.));
#21659=CARTESIAN_POINT('',(463.5,-261.,-469.));
#21660=CARTESIAN_POINT('',(463.5,-276.875,-469.));
#21661=CARTESIAN_POINT('Origin',(0.,-276.875,-3.24206954336256E-14));
#21662=CARTESIAN_POINT('Origin',(0.,-261.,-3.08921332011904E-14));
#21663=CARTESIAN_POINT('Origin',(-463.5,-276.875,-5.17905770564469E-14));
#21664=CARTESIAN_POINT('',(-463.5,-261.,-469.));
#21665=CARTESIAN_POINT('',(-463.5,-261.,-5.02620148240116E-14));
#21666=CARTESIAN_POINT('',(-463.5,-261.,-5.02620148240116E-14));
#21667=CARTESIAN_POINT('',(-463.5,-276.875,-469.));
#21668=CARTESIAN_POINT('',(-463.5,-276.875,-469.));
#21669=CARTESIAN_POINT('',(-463.5,-276.875,-5.17905770564469E-14));
#21670=CARTESIAN_POINT('',(-463.5,-276.875,-5.17905770564469E-14));
#21671=CARTESIAN_POINT('',(-463.5,-276.875,-5.17905770564469E-14));
#21672=CARTESIAN_POINT('Origin',(-463.5,-276.875,-5.17905770564469E-14));
#21673=CARTESIAN_POINT('',(-412.7,-261.,-3.13522131516744E-14));
#21674=CARTESIAN_POINT('',(-463.5,-261.,-5.02620148240116E-14));
#21675=CARTESIAN_POINT('',(-412.7,-276.875,-3.28807753841096E-14));
#21676=CARTESIAN_POINT('',(-463.5,-276.875,-5.17905770564469E-14));
#21677=CARTESIAN_POINT('',(-412.7,-276.875,-3.28807753841096E-14));
#21678=CARTESIAN_POINT('Origin',(-412.7,-276.875,-3.28807753841096E-14));
#21679=CARTESIAN_POINT('',(-412.7,-261.,-469.));
#21680=CARTESIAN_POINT('',(-412.7,-261.,-3.13522131516744E-14));
#21681=CARTESIAN_POINT('',(-412.7,-276.875,-469.));
#21682=CARTESIAN_POINT('',(-412.7,-276.875,-3.28807753841096E-14));
#21683=CARTESIAN_POINT('',(-412.7,-276.875,-469.));
#21684=CARTESIAN_POINT('Origin',(-463.5,-276.875,-469.));
#21685=CARTESIAN_POINT('',(-463.5,-261.,-469.));
#21686=CARTESIAN_POINT('',(-463.5,-276.875,-469.));
#21687=CARTESIAN_POINT('Origin',(0.,-276.875,-3.24206954336256E-14));
#21688=CARTESIAN_POINT('Origin',(0.,-261.,-3.08921332011904E-14));
#32871=UNCERTAINTY_MEASURE_WITH_UNIT(LENGTH_MEASURE(0.01),#32904,
'DISTANCE_ACCURACY_VALUE',
'Maximum model space distance between geometric entities at asserted c
onnectivities');
#32886=UNCERTAINTY_MEASURE_WITH_UNIT(LENGTH_MEASURE(0.01),#32904,
'DISTANCE_ACCURACY_VALUE',
'Maximum model space distance between geometric entities at asserted c
onnectivities');
#32888=(
GEOMETRIC_REPRESENTATION_CONTEXT(3)
GLOBAL_UNCERTAINTY_ASSIGNED_CONTEXT((#32871))
GLOBAL_UNIT_ASSIGNED_CONTEXT((#32904,#32906,#32907))
REPRESENTATION_CONTEXT('','3D')
);
#32903=(
GEOMETRIC_REPRESENTATION_CONTEXT(3)
GLOBAL_UNCERTAINTY_ASSIGNED_CONTEXT((#32886))
GLOBAL_UNIT_ASSIGNED_CONTEXT((#32904,#32906,#32907))
REPRESENTATION_CONTEXT('','3D')
);
#32904=(
LENGTH_UNIT()
NAMED_UNIT(*)
SI_UNIT(.MILLI.,.METRE.)
);
#32906=(
NAMED_UNIT(*)
PLANE_ANGLE_UNIT()
SI_UNIT($,.RADIAN.)
);
#32907=(
NAMED_UNIT(*)
SI_UNIT($,.STERADIAN.)
SOLID_ANGLE_UNIT()
);
#32909=SHAPE_DEFINITION_REPRESENTATION(#32925,#33013);
#32925=PRODUCT_DEFINITION_SHAPE('',$,#33030);
#33013=SHAPE_REPRESENTATION('',(#15784),#32888);
#33028=PRODUCT_DEFINITION_CONTEXT('part definition',#33078,'design');
#33030=PRODUCT_DEFINITION('Head Compartment','Head Compartment',#33046,
#33028);
#33046=PRODUCT_DEFINITION_FORMATION('',$,#33081);
#33078=APPLICATION_CONTEXT(
'Core Data for Automotive Mechanical Design Process');
#33079=PRODUCT_CONTEXT('part definition',#33078,'mechanical');
#33081=PRODUCT('Head Compartment','Head Compartment',$,(#33079));
#33097=PRESENTATION_STYLE_ASSIGNMENT((#33103));
#33103=SURFACE_STYLE_USAGE(.BOTH.,#33109);
#33109=SURFACE_SIDE_STYLE('',(#33115));
#33115=SURFACE_STYLE_FILL_AREA(#33121);
#33121=FILL_AREA_STYLE('Opaque(61,176,222)',(#33127));
#33127=FILL_AREA_STYLE_COLOUR('Opaque(61,176,222)',#33133);
#33133=COLOUR_RGB('Opaque(61,176,222)',0.23921568627451,0.690196078431373,
0.870588235294118);
ENDSEC;
END-ISO-10303-21;
